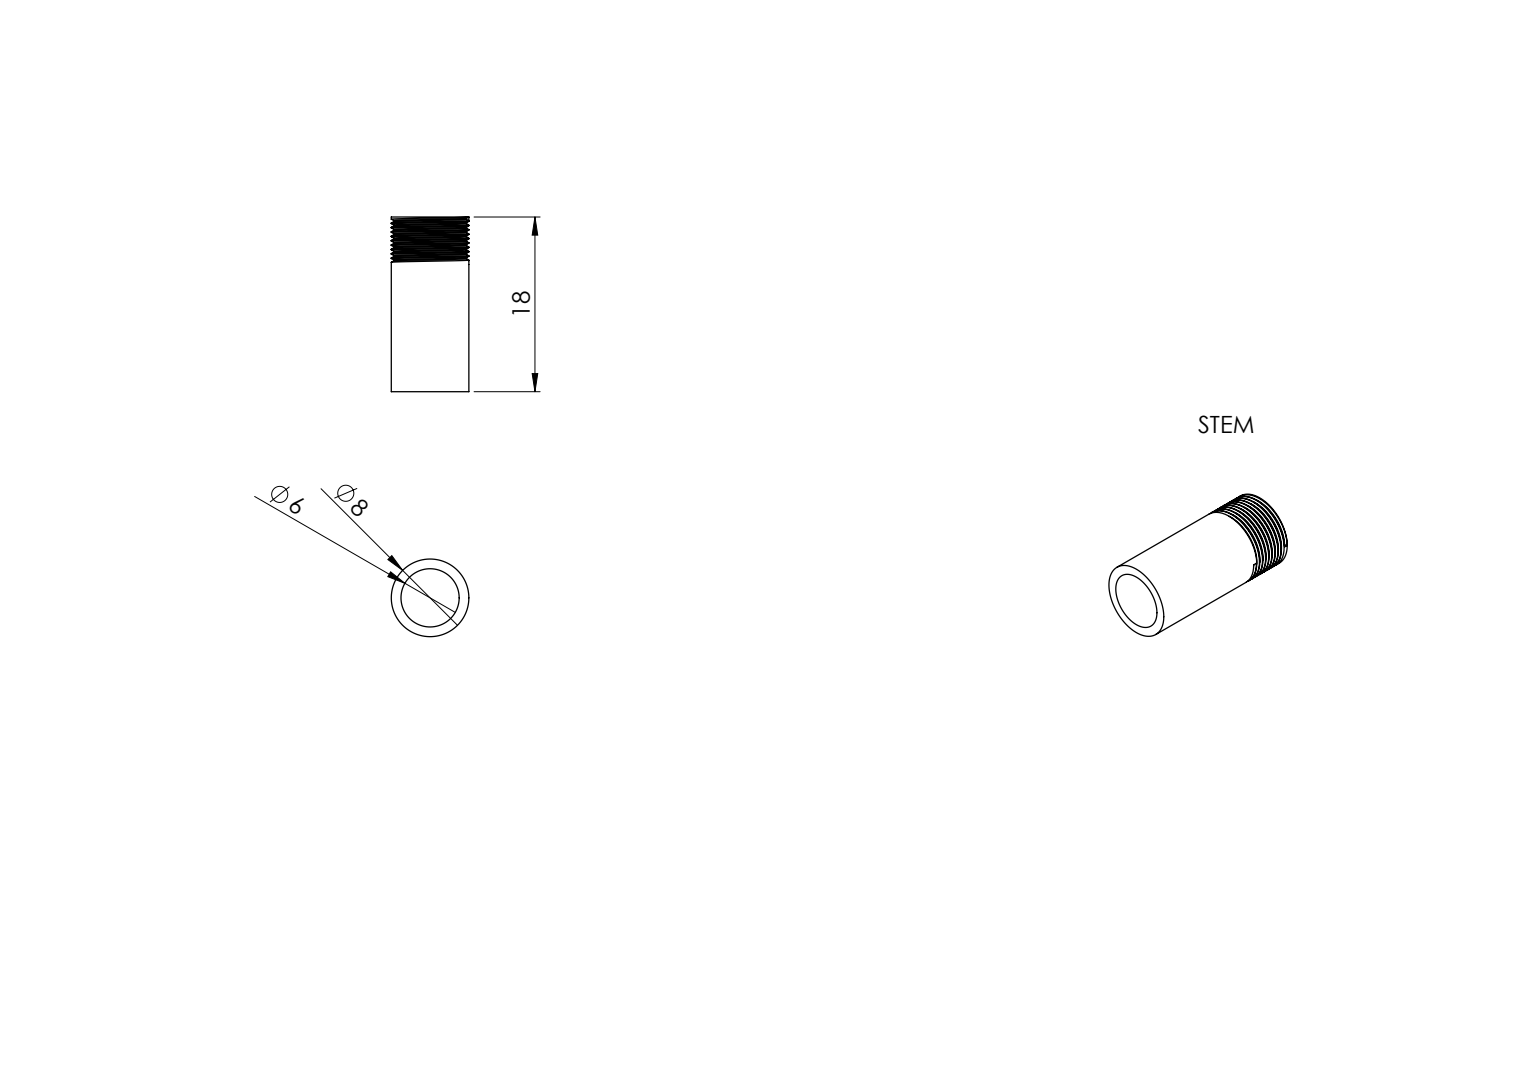
ISO-10303-21;
HEADER;
FILE_DESCRIPTION (('STEP AP214'),
    '1' );
FILE_NAME ('stem.step',
    '2026-10-26T12:50:16',
    ( '' ),
    ( '' ),
    'SwSTEP 2.0',
    'SolidWorks 2026',
    '' );
FILE_SCHEMA (( 'AUTOMOTIVE_DESIGN' ));
ENDSEC;

DATA;
#2=CARTESIAN_POINT ( 'NONE',  ( -3.756430356249997882, -11.16877607737301226, 2.653124999385483296 ) ) ;
#3=CARTESIAN_POINT ( 'NONE',  ( 2.000000000000003997, -5.535898384862238508, 4.518749998770967835 ) ) ;
#8=CARTESIAN_POINT ( 'NONE',  ( 4.000000000000003553, -8.999999999999992895, 1.743749998770967924 ) ) ;
#9=CARTESIAN_POINT ( 'NONE',  ( 2.620986760973688460E-15, -13.61880215351699874, 3.037499999999999201 ) ) ;
#11=CARTESIAN_POINT ( 'NONE',  ( 4.000000000000003553, -8.999999999999992895, 2.643749998770966059 ) ) ;
#36=CARTESIAN_POINT ( 'NONE',  ( 3.756430356250004099, -6.831223922626973533, 1.190624999385485383 ) ) ;
#74=( BOUNDED_CURVE ( )  B_SPLINE_CURVE ( 2, ( #2295, #21785, #5959, #10252, #8301, #13672, #11709 ),
 .UNSPECIFIED., .F., .F. ) 
 B_SPLINE_CURVE_WITH_KNOTS ( ( 3, 2, 2, 3 ),
 ( 0.8999999999999996891, 0.9166666666666665186, 0.9333333333333335702, 0.9500000000000003997 ),
 .UNSPECIFIED. ) 
 CURVE ( )  GEOMETRIC_REPRESENTATION_ITEM ( )  RATIONAL_B_SPLINE_CURVE ( ( 1.000000000000002665, 0.8660254037844360431, 1.000000000000000000, 0.8660254037844387076, 1.000000000000000000, 0.8660254037844351549, 1.000000000000003553 ) ) 
 REPRESENTATION_ITEM ( '' )  );
#103=CARTESIAN_POINT ( 'NONE',  ( 2.672651547586948120E-15, -13.33755215474603162, 2.278124999385481964 ) ) ;
#109=SHAPE_REPRESENTATION_RELATIONSHIP ( 'NONE' , 'NONE' ,  #19829, #5978 ) ;
#141=CARTESIAN_POINT ( 'NONE',  ( -3.756430356249997882, -11.16877607737301226, 4.453124999385482674 ) ) ;
#142=CARTESIAN_POINT ( 'NONE',  ( 1.878215178125004048, -5.746835883940462963, 0.3281249993854831737 ) ) ;
#162=EDGE_LOOP ( 'NONE', ( #20423, #8282, #5140, #7710 ) ) ;
#171=CARTESIAN_POINT ( 'NONE',  ( 1.878215178125000939, -12.25316411605952283, 3.778124999385484628 ) ) ;
#176=CARTESIAN_POINT ( 'NONE',  ( 3.756430356250003655, -8.999999999999992895, 0.5906249993854819635 ) ) ;
#227=CARTESIAN_POINT ( 'NONE',  ( -3.756430356249996994, -8.999999999999992895, 3.515624999385482674 ) ) ;
#266=CARTESIAN_POINT ( 'NONE',  ( -1.999999999999995781, -5.535898384862237620, 4.593749998770966236 ) ) ;
#277=ADVANCED_FACE ( 'NONE', ( #3080 ), #9085, .T. ) ;
#279=CARTESIAN_POINT ( 'NONE',  ( 3.999999999999994227, -11.30940107675849937, 1.762499999999997735 ) ) ;
#293=CARTESIAN_POINT ( 'NONE',  ( -3.756430356249996994, -8.999999999999992895, 2.728124999385482585 ) ) ;
#294=CARTESIAN_POINT ( 'NONE',  ( -1.999999999999995781, -5.535898384862237620, 1.443749998770966325 ) ) ;
#298=CARTESIAN_POINT ( 'NONE',  ( 1.878215178125000939, -12.25316411605952283, 0.9656249993854824076 ) ) ;
#337=VERTEX_POINT ( 'NONE', #16684 ) ;
#344=EDGE_CURVE ( 'NONE', #1313, #21005, #7390, .T. ) ;
#350=CARTESIAN_POINT ( 'NONE',  ( 1.878215178125000939, -12.25316411605952283, 4.565624999385481608 ) ) ;
#353=CARTESIAN_POINT ( 'NONE',  ( 3.752267015613588906E-15, -4.381197846482986158, 1.012499999999998401 ) ) ;
#392=CARTESIAN_POINT ( 'NONE',  ( 3.735045420075836212E-15, -4.662447845253954171, 2.165624999385483029 ) ) ;
#404=CARTESIAN_POINT ( 'NONE',  ( 4.000000000000003553, -8.999999999999992895, 2.700000000000001066 ) ) ;
#428=CARTESIAN_POINT ( 'NONE',  ( 3.756430356250002323, -11.16877607737301226, 1.565624999385482941 ) ) ;
#429=CARTESIAN_POINT ( 'NONE',  ( -4.000000000000033751, -6.690598923241509510, 1.481249998770963749 ) ) ;
#434=CARTESIAN_POINT ( 'NONE',  ( 1.878215178125004048, -5.746835883940462963, 1.565624999385482274 ) ) ;
#435=CARTESIAN_POINT ( 'NONE',  ( 2.000000000000003997, -5.535898384862238508, 3.675000000000001155 ) ) ;
#439=CARTESIAN_POINT ( 'NONE',  ( -1.878215178124998497, -12.25316411605951927, 1.003124999385485161 ) ) ;
#466=EDGE_CURVE ( 'NONE', #13776, #14884, #16423, .T. ) ;
#470=CARTESIAN_POINT ( 'NONE',  ( 4.000000000000003553, -8.999999999999992895, 0.1968749993854837510 ) ) ;
#523=VERTEX_POINT ( 'NONE', #23469 ) ;
#526=CARTESIAN_POINT ( 'NONE',  ( -1.999999999999995781, -5.535898384862237620, 1.950000000000000400 ) ) ;
#528=CARTESIAN_POINT ( 'NONE',  ( -3.756430356249997882, -11.16877607737301226, 3.215624999385481964 ) ) ;
#543=DIRECTION ( 'NONE',  ( 0.000000000000000000, 0.000000000000000000, 1.000000000000000000 ) ) ;
#561=CARTESIAN_POINT ( 'NONE',  ( -1.878215178124998497, -12.25316411605951927, 2.353124999385485694 ) ) ;
#568=CARTESIAN_POINT ( 'NONE',  ( 3.756430356250004099, -6.831223922626973533, 2.428124999385481431 ) ) ;
#573=CARTESIAN_POINT ( 'NONE',  ( -1.878215178124998497, -12.25316411605951927, 1.453124999385484228 ) ) ;
#574=FACE_OUTER_BOUND ( 'NONE', #3616, .T. ) ;
#586=CARTESIAN_POINT ( 'NONE',  ( 3.756430356250003655, -8.999999999999992895, 4.640624999385483562 ) ) ;
#651=CARTESIAN_POINT ( 'NONE',  ( 4.000000000000032863, -11.30940107675847983, 3.506249998770968102 ) ) ;
#652=CARTESIAN_POINT ( 'NONE',  ( 1.878215178125004048, -5.746835883940462963, 1.228124999385484584 ) ) ;
#668=CARTESIAN_POINT ( 'NONE',  ( -3.999999999999995559, -6.690598923241487306, 3.731249998770965970 ) ) ;
#669=ORIENTED_EDGE ( 'NONE', *, *, #3778, .F. ) ;
#677=ORIENTED_EDGE ( 'NONE', *, *, #7902, .T. ) ;
#682=CARTESIAN_POINT ( 'NONE',  ( 3.756430356250004099, -6.831223922626973533, 3.440624999385483829 ) ) ;
#686=DIRECTION ( 'NONE',  ( -0.000000000000000000, -0.000000000000000000, -1.000000000000000000 ) ) ;
#687=CARTESIAN_POINT ( 'NONE',  ( -3.999999999999953371, -6.690598923241463325, 0.6374999999999958478 ) ) ;
#689=CARTESIAN_POINT ( 'NONE',  ( -1.878215178124998497, -12.25316411605951927, 0.8906249993854836733 ) ) ;
#694=CARTESIAN_POINT ( 'NONE',  ( -1.878215178124995832, -5.746835883940462963, 2.653124999385483740 ) ) ;
#702=VERTEX_POINT ( 'NONE', #9421 ) ;
#705=ORIENTED_EDGE ( 'NONE', *, *, #13948, .T. ) ;
#737=CARTESIAN_POINT ( 'NONE',  ( -3.999999999999996447, -8.999999999999992895, 1.125000000000000888 ) ) ;
#768=ADVANCED_FACE ( 'NONE', ( #3150 ), #24982, .T. ) ;
#770=CARTESIAN_POINT ( 'NONE',  ( -3.756430356249995661, -6.831223922626973533, 0.8906249993854814528 ) ) ;
#776=CARTESIAN_POINT ( 'NONE',  ( 3.469446951953614189E-15, -8.999999999999992895, 18.00000000000000000 ) ) ;
#792=AXIS2_PLACEMENT_3D ( 'NONE', #15459, #16816, #19491 ) ;
#798=DIRECTION ( 'NONE',  ( -0.000000000000000000, -0.000000000000000000, -1.000000000000000000 ) ) ;
#801=CARTESIAN_POINT ( 'NONE',  ( 2.672651547586948120E-15, -13.33755215474602984, 4.640624999385483562 ) ) ;
#808=CARTESIAN_POINT ( 'NONE',  ( -1.878215178124995832, -5.746835883940462963, 3.890624999385482674 ) ) ;
#811=CARTESIAN_POINT ( 'NONE',  ( -1.999999999999995781, -5.535898384862237620, 3.750000000000000000 ) ) ;
#814=CARTESIAN_POINT ( 'NONE',  ( -3.756430356249996105, -6.831223922626973533, 3.140624999385484006 ) ) ;
#834=AXIS2_PLACEMENT_3D ( 'NONE', #5383, #9320, #12752 ) ;
#856=ORIENTED_EDGE ( 'NONE', *, *, #17515, .T. ) ;
#860=CARTESIAN_POINT ( 'NONE',  ( 3.999999999999956035, -11.30940107675852602, 4.406249998770962684 ) ) ;
#861=ORIENTED_EDGE ( 'NONE', *, *, #11086, .T. ) ;
#908=CARTESIAN_POINT ( 'NONE',  ( -3.756430356249995661, -6.831223922626973533, 1.790624999385484806 ) ) ;
#917=DIRECTION ( 'NONE',  ( 0.8660254037844397068, 0.000000000000000000, -0.4999999999999983347 ) ) ;
#921=LINE ( 'NONE', #7050, #24021 ) ;
#927=ORIENTED_EDGE ( 'NONE', *, *, #22382, .F. ) ;
#934=ORIENTED_EDGE ( 'NONE', *, *, #15408, .T. ) ;
#945=CARTESIAN_POINT ( 'NONE',  ( -3.756430356249996994, -8.999999999999992895, 0.3656249993854825409 ) ) ;
#951=CARTESIAN_POINT ( 'NONE',  ( 1.878215178125004048, -5.746835883940462963, 3.365624999385481875 ) ) ;
#953=CARTESIAN_POINT ( 'NONE',  ( -3.999999999999997335, -11.30940107675849404, 3.862499999999996714 ) ) ;
#988=CARTESIAN_POINT ( 'NONE',  ( 3.756430356250004099, -6.831223922626973533, 0.1781249993854828739 ) ) ;
#1034=CARTESIAN_POINT ( 'NONE',  ( -1.878215178124995832, -5.746835883940462963, 4.003124999385484273 ) ) ;
#1065=CARTESIAN_POINT ( 'NONE',  ( 3.756430356250002323, -11.16877607737301226, 0.5531249993854806535 ) ) ;
#1070=CARTESIAN_POINT ( 'NONE',  ( 2.620986760973688460E-15, -13.61880215351699874, 0.3375000000000008549 ) ) ;
#1074=DIRECTION ( 'NONE',  ( 0.000000000000000000, 0.000000000000000000, -1.000000000000000000 ) ) ;
#1075=CARTESIAN_POINT ( 'NONE',  ( -1.878215178124995832, -5.746835883940462963, 4.453124999385483562 ) ) ;
#1079=ORIENTED_EDGE ( 'NONE', *, *, #19912, .F. ) ;
#1091=DIRECTION ( 'NONE',  ( -0.000000000000000000, -0.000000000000000000, -1.000000000000000000 ) ) ;
#1108=EDGE_LOOP ( 'NONE', ( #16463, #25740, #25010, #7826 ) ) ;
#1148=CARTESIAN_POINT ( 'NONE',  ( -3.756430356249997438, -11.16877607737301048, 0.8531249993854844726 ) ) ;
#1155=LINE ( 'NONE', #20782, #4194 ) ;
#1181=CARTESIAN_POINT ( 'NONE',  ( 1.878215178125004048, -5.746835883940462963, 4.378124999385484273 ) ) ;
#1182=CARTESIAN_POINT ( 'NONE',  ( 2.000000000000003997, -5.535898384862238508, 1.818749998770966769 ) ) ;
#1188=CARTESIAN_POINT ( 'NONE',  ( 3.756430356250002323, -11.16877607737301226, 4.603124999385482141 ) ) ;
#1194=CARTESIAN_POINT ( 'NONE',  ( 3.756430356250003211, -6.831223922626973533, 3.890624999385483562 ) ) ;
#1197=VECTOR ( 'NONE', #3668, 1000.000000000000000 ) ;
#1201=ORIENTED_EDGE ( 'NONE', *, *, #18891, .T. ) ;
#1209=( BOUNDED_CURVE ( )  B_SPLINE_CURVE ( 2, ( #19108, #17166, #3281, #7221, #15205, #23173, #11254 ),
 .UNSPECIFIED., .F., .F. ) 
 B_SPLINE_CURVE_WITH_KNOTS ( ( 3, 2, 2, 3 ),
 ( 0.000000000000000000, 0.01666666666666663521, 0.03333333333333327042, 0.04999999999999990563 ),
 .UNSPECIFIED. ) 
 CURVE ( )  GEOMETRIC_REPRESENTATION_ITEM ( )  RATIONAL_B_SPLINE_CURVE ( ( 1.000000000000000000, 0.8660254037844387076, 1.000000000000000000, 0.8660254037844387076, 1.000000000000000000, 0.8660254037844394848, 0.9999999999999992228 ) ) 
 REPRESENTATION_ITEM ( '' )  );
#1218=VECTOR ( 'NONE', #19343, 1000.000000000000000 ) ;
#1283=CARTESIAN_POINT ( 'NONE',  ( -3.756430356249996105, -6.831223922626973533, 0.7781249993854825187 ) ) ;
#1285=AXIS2_PLACEMENT_3D ( 'NONE', #1608, #11806, #20026 ) ;
#1313=VERTEX_POINT ( 'NONE', #11561 ) ;
#1323=CARTESIAN_POINT ( 'NONE',  ( 1.878215178125004048, -5.746835883940462963, 1.565624999385482274 ) ) ;
#1324=CARTESIAN_POINT ( 'NONE',  ( -1.999999999999995781, -5.535898384862237620, 1.443749998770966325 ) ) ;
#1332=CARTESIAN_POINT ( 'NONE',  ( -1.878215178124995832, -5.746835883940462963, 2.990624999385481431 ) ) ;
#1334=LINE ( 'NONE', #11391, #10437 ) ;
#1340=CARTESIAN_POINT ( 'NONE',  ( 3.756430356250003211, -6.831223922626973533, 3.440624999385483829 ) ) ;
#1403=CARTESIAN_POINT ( 'NONE',  ( 4.000000000000003553, -8.999999999999992895, 3.093749998770968457 ) ) ;
#1417=EDGE_LOOP ( 'NONE', ( #18226, #25662, #5734, #10746 ) ) ;
#1420=CARTESIAN_POINT ( 'NONE',  ( 3.735045420075836212E-15, -4.662447845253954171, 2.053124999385483651 ) ) ;
#1422=ADVANCED_FACE ( 'NONE', ( #24079 ), #8392, .F. ) ;
#1445=VERTEX_POINT ( 'NONE', #14802 ) ;
#1453=CARTESIAN_POINT ( 'NONE',  ( -3.756430356249995661, -6.831223922626973533, 2.578124999385481342 ) ) ;
#1454=CARTESIAN_POINT ( 'NONE',  ( 4.000000000000003553, -8.999999999999992895, 2.643749998770966059 ) ) ;
#1459=CARTESIAN_POINT ( 'NONE',  ( 2.000000000000000888, -12.46410161513774817, 2.174999999999999822 ) ) ;
#1464=CARTESIAN_POINT ( 'NONE',  ( 2.672651547586948120E-15, -13.33755215474603162, 4.190624999385483385 ) ) ;
#1485=CARTESIAN_POINT ( 'NONE',  ( 3.469446951953614189E-15, -8.999999999999992895, 18.00000000000000000 ) ) ;
#1502=CARTESIAN_POINT ( 'NONE',  ( 4.000000000000049738, -6.690598923241514839, 4.087499999999997691 ) ) ;
#1536=EDGE_CURVE ( 'NONE', #4330, #17764, #6946, .T. ) ;
#1542=CARTESIAN_POINT ( 'NONE',  ( 3.735045420075836212E-15, -4.662447845253954171, 3.965624999385486404 ) ) ;
#1558=ORIENTED_EDGE ( 'NONE', *, *, #2307, .F. ) ;
#1572=CARTESIAN_POINT ( 'NONE',  ( 1.878215178125004048, -5.746835883940462963, 2.015624999385484450 ) ) ;
#1573=CARTESIAN_POINT ( 'NONE',  ( 2.620986760973688460E-15, -13.61880215351699874, 1.181249998770967258 ) ) ;
#1578=CARTESIAN_POINT ( 'NONE',  ( 4.000000000000003553, -8.999999999999992895, 1.799999999999999600 ) ) ;
#1589=CARTESIAN_POINT ( 'NONE',  ( 4.000000000000003553, -8.999999999999992895, 3.993749998770966592 ) ) ;
#1608=CARTESIAN_POINT ( 'NONE',  ( 3.469446951953614189E-15, -8.999999999999992895, 18.00000000000000000 ) ) ;
#1670=CARTESIAN_POINT ( 'NONE',  ( -3.756430356249997438, -11.16877607737301048, 0.4031249993854806868 ) ) ;
#1688=EDGE_CURVE ( 'NONE', #1445, #19775, #10234, .T. ) ;
#1689=CARTESIAN_POINT ( 'NONE',  ( 4.000000000000034639, -6.690598923241508622, 2.287499999999995648 ) ) ;
#1691=DIRECTION ( 'NONE',  ( 0.000000000000000000, 0.000000000000000000, 1.000000000000000000 ) ) ;
#1710=CARTESIAN_POINT ( 'NONE',  ( -3.756430356249996994, -8.999999999999992895, 3.965624999385481519 ) ) ;
#1711=CARTESIAN_POINT ( 'NONE',  ( -1.999999999999995781, -5.535898384862237620, 0.9937499987709673688 ) ) ;
#1717=CARTESIAN_POINT ( 'NONE',  ( 4.000000000000003553, -6.690598923241489970, 1.387499999999999956 ) ) ;
#1747=CARTESIAN_POINT ( 'NONE',  ( 3.469446951953614189E-15, -8.999999999999992895, 18.00000000000000000 ) ) ;
#1756=CARTESIAN_POINT ( 'NONE',  ( -1.878215178124995832, -5.746835883940462963, 0.4031249993854852942 ) ) ;
#1770=VERTEX_POINT ( 'NONE', #6410 ) ;
#1772=CARTESIAN_POINT ( 'NONE',  ( -4.000000000000057732, -6.690598923241522833, 4.237499999999998934 ) ) ;
#1792=ORIENTED_EDGE ( 'NONE', *, *, #11977, .T. ) ;
#1808=CARTESIAN_POINT ( 'NONE',  ( 1.878215178125004048, -5.746835883940462963, 2.915624999385482585 ) ) ;
#1839=EDGE_CURVE ( 'NONE', #12074, #6033, #921, .T. ) ;
#1845=CARTESIAN_POINT ( 'NONE',  ( -3.756430356249995661, -6.831223922626973533, 3.478124999385480809 ) ) ;
#1846=CARTESIAN_POINT ( 'NONE',  ( 3.735045420075836212E-15, -4.662447845253954171, 0.8156249993854834957 ) ) ;
#1851=CARTESIAN_POINT ( 'NONE',  ( 3.752267015613588906E-15, -4.381197846482986158, 2.362499999999997602 ) ) ;
#1861=DIRECTION ( 'NONE',  ( 0.000000000000000000, 0.000000000000000000, -1.000000000000000000 ) ) ;
#1864=DIRECTION ( 'NONE',  ( 1.000000000000000000, 0.000000000000000000, 0.000000000000000000 ) ) ;
#1875=CARTESIAN_POINT ( 'NONE',  ( 3.735045420075836212E-15, -4.662447845253954171, 0.3656249993854837066 ) ) ;
#1893=ORIENTED_EDGE ( 'NONE', *, *, #23260, .F. ) ;
#1904=( BOUNDED_CURVE ( )  B_SPLINE_CURVE ( 2, ( #10676, #20494, #20632, #22333, #12389, #4415, #20108 ),
 .UNSPECIFIED., .F., .F. ) 
 B_SPLINE_CURVE_WITH_KNOTS ( ( 3, 2, 2, 3 ),
 ( 0.2500000000000002776, 0.2666666666666669405, 0.2833333333333335480, 0.3000000000000002109 ),
 .UNSPECIFIED. ) 
 CURVE ( )  GEOMETRIC_REPRESENTATION_ITEM ( )  RATIONAL_B_SPLINE_CURVE ( ( 0.9999999999999977796, 0.8660254037844409281, 1.000000000000000000, 0.8660254037844387076, 1.000000000000000000, 0.8660254037844369313, 1.000000000000001776 ) ) 
 REPRESENTATION_ITEM ( '' )  );
#1929=CARTESIAN_POINT ( 'NONE',  ( 3.756430356250003211, -6.831223922626973533, 4.228124999385484806 ) ) ;
#1932=CARTESIAN_POINT ( 'NONE',  ( -4.000000000000012434, -11.30940107675848516, 3.862499999999996714 ) ) ;
#1960=CARTESIAN_POINT ( 'NONE',  ( 3.756430356250004099, -6.831223922626973533, 3.778124999385480631 ) ) ;
#1961=CARTESIAN_POINT ( 'NONE',  ( 2.000000000000000888, -12.46410161513774817, 3.468749998770968901 ) ) ;
#1967=CARTESIAN_POINT ( 'NONE',  ( 4.000000000000003553, -8.999999999999992895, 1.350000000000000533 ) ) ;
#1978=CARTESIAN_POINT ( 'NONE',  ( 4.000000000000003553, -8.999999999999992895, 4.696874999385483918 ) ) ;
#1990=CARTESIAN_POINT ( 'NONE',  ( 1.878215178125000939, -12.25316411605952283, 1.078124999385483784 ) ) ;
#2046=DIRECTION ( 'NONE',  ( -0.000000000000000000, -0.000000000000000000, -1.000000000000000000 ) ) ;
#2051=( BOUNDED_CURVE ( )  B_SPLINE_CURVE ( 2, ( #6648, #14634, #22615, #4703, #10569, #651, #16728 ),
 .UNSPECIFIED., .F., .F. ) 
 B_SPLINE_CURVE_WITH_KNOTS ( ( 3, 2, 2, 3 ),
 ( 0.6500000000000002442, 0.6666666666666668517, 0.6833333333333335702, 0.7000000000000001776 ),
 .UNSPECIFIED. ) 
 CURVE ( )  GEOMETRIC_REPRESENTATION_ITEM ( )  RATIONAL_B_SPLINE_CURVE ( ( 0.9999999999999982236, 0.8660254037844404840, 1.000000000000000000, 0.8660254037844387076, 1.000000000000000000, 0.8660254037844369313, 1.000000000000001776 ) ) 
 REPRESENTATION_ITEM ( '' )  );
#2053=VECTOR ( 'NONE', #21376, 1000.000000000000000 ) ;
#2055=CARTESIAN_POINT ( 'NONE',  ( 3.756430356250002323, -11.16877607737301403, 4.153124999385482852 ) ) ;
#2059=CARTESIAN_POINT ( 'NONE',  ( 2.620986760973688460E-15, -13.61880215351699874, 3.937499999999998224 ) ) ;
#2070=CARTESIAN_POINT ( 'NONE',  ( -1.999999999999995781, -5.535898384862237620, 2.399999999999999467 ) ) ;
#2091=CARTESIAN_POINT ( 'NONE',  ( 1.878215178125000939, -12.25316411605952283, 4.115624999385482319 ) ) ;
#2092=CARTESIAN_POINT ( 'NONE',  ( -1.999999999999998224, -12.46410161513774639, 4.293749998770968190 ) ) ;
#2104=VECTOR ( 'NONE', #14071, 1000.000000000000000 ) ;
#2114=CYLINDRICAL_SURFACE ( 'NONE', #6645, 4.000000000000000000 ) ;
#2118=CARTESIAN_POINT ( 'NONE',  ( 2.000000000000003997, -5.535898384862238508, 2.718749998770968013 ) ) ;
#2134=CARTESIAN_POINT ( 'NONE',  ( -1.878215178124998497, -12.25316411605951927, 1.790624999385481697 ) ) ;
#2142=ORIENTED_EDGE ( 'NONE', *, *, #19912, .T. ) ;
#2148=CARTESIAN_POINT ( 'NONE',  ( 4.000000000000003553, -8.999999999999992895, 0.3937499987709675020 ) ) ;
#2174=LINE ( 'NONE', #10135, #11663 ) ;
#2191=CARTESIAN_POINT ( 'NONE',  ( -1.878215178124995832, -5.746835883940462963, 2.090624999385483296 ) ) ;
#2196=CARTESIAN_POINT ( 'NONE',  ( 3.999999999999956035, -11.30940107675852602, 4.012499999999995737 ) ) ;
#2225=EDGE_CURVE ( 'NONE', #11292, #18617, #20028, .T. ) ;
#2227=CARTESIAN_POINT ( 'NONE',  ( -1.878215178124995832, -5.746835883940462963, 4.340624999385481964 ) ) ;
#2228=CARTESIAN_POINT ( 'NONE',  ( -1.999999999999995781, -5.535898384862237620, 3.693749998770968546 ) ) ;
#2258=CARTESIAN_POINT ( 'NONE',  ( 3.756430356250002323, -11.16877607737301226, 2.015624999385483118 ) ) ;
#2264=CARTESIAN_POINT ( 'NONE',  ( 3.756430356250003655, -8.999999999999992895, 2.390624999385481342 ) ) ;
#2267=CARTESIAN_POINT ( 'NONE',  ( 3.469446951953614189E-15, -8.999999999999992895, 0.000000000000000000 ) ) ;
#2270=FACE_OUTER_BOUND ( 'NONE', #11908, .T. ) ;
#2276=ORIENTED_EDGE ( 'NONE', *, *, #7804, .F. ) ;
#2295=CARTESIAN_POINT ( 'NONE',  ( 4.000000000000003553, -8.999999999999992895, 4.443749998770965881 ) ) ;
#2307=EDGE_CURVE ( 'NONE', #20603, #13396, #13885, .T. ) ;
#2315=CARTESIAN_POINT ( 'NONE',  ( 3.756430356250003211, -6.831223922626973533, 3.778124999385480631 ) ) ;
#2332=ORIENTED_EDGE ( 'NONE', *, *, #22414, .T. ) ;
#2342=PRODUCT_DEFINITION_SHAPE ( 'NONE', 'NONE',  #17659 ) ;
#2348=CARTESIAN_POINT ( 'NONE',  ( 2.672651547586948120E-15, -13.33755215474602984, 4.078124999385480010 ) ) ;
#2349=CARTESIAN_POINT ( 'NONE',  ( 3.756430356250003655, -8.999999999999992895, 0.7031249993854835623 ) ) ;
#2360=CARTESIAN_POINT ( 'NONE',  ( 3.999999999999942268, -6.690598923241455331, 2.737500000000000266 ) ) ;
#2372=VERTEX_POINT ( 'NONE', #20006 ) ;
#2379=CARTESIAN_POINT ( 'NONE',  ( 3.735045420075836212E-15, -4.662447845253954171, 2.615624999385482319 ) ) ;
#2380=CARTESIAN_POINT ( 'NONE',  ( 3.752267015613588906E-15, -4.381197846482986158, 1.406249998770964904 ) ) ;
#2384=CARTESIAN_POINT ( 'NONE',  ( 3.756430356250002323, -11.16877607737301226, 1.003124999385480276 ) ) ;
#2387=CARTESIAN_POINT ( 'NONE',  ( 3.756430356250002323, -11.16877607737301403, 2.015624999385483118 ) ) ;
#2426=ORIENTED_EDGE ( 'NONE', *, *, #22750, .F. ) ;
#2458=ORIENTED_EDGE ( 'NONE', *, *, #23613, .T. ) ;
#2467=CARTESIAN_POINT ( 'NONE',  ( 3.756430356250004099, -6.831223922626973533, 2.540624999385480809 ) ) ;
#2490=ORIENTED_EDGE ( 'NONE', *, *, #11535, .T. ) ;
#2500=ORIENTED_EDGE ( 'NONE', *, *, #20767, .T. ) ;
#2506=CARTESIAN_POINT ( 'NONE',  ( 3.756430356250004099, -6.831223922626973533, 2.540624999385480809 ) ) ;
#2512=CARTESIAN_POINT ( 'NONE',  ( 1.878215178125004048, -5.746835883940462963, 2.015624999385484450 ) ) ;
#2516=CARTESIAN_POINT ( 'NONE',  ( -3.756430356249996105, -6.831223922626973533, 0.8906249993854813418 ) ) ;
#2518=DIRECTION ( 'NONE',  ( -0.000000000000000000, -0.000000000000000000, -1.000000000000000000 ) ) ;
#2545=CARTESIAN_POINT ( 'NONE',  ( -3.999999999999996447, -8.999999999999992895, 2.024999999999999023 ) ) ;
#2589=EDGE_CURVE ( 'NONE', #13396, #21005, #14278, .T. ) ;
#2612=CARTESIAN_POINT ( 'NONE',  ( 1.878215178125000939, -12.25316411605952283, 1.978124999385485250 ) ) ;
#2620=CARTESIAN_POINT ( 'NONE',  ( -3.999999999999953371, -6.690598923241463325, 1.031249998770966458 ) ) ;
#2623=CARTESIAN_POINT ( 'NONE',  ( 4.000000000000003553, -8.999999999999992895, 3.149999999999999911 ) ) ;
#2644=CARTESIAN_POINT ( 'NONE',  ( -1.878215178124995832, -5.746835883940462963, 3.103124999385483029 ) ) ;
#2649=CARTESIAN_POINT ( 'NONE',  ( 1.878215178125004048, -5.746835883940462963, 2.915624999385482585 ) ) ;
#2651=CARTESIAN_POINT ( 'NONE',  ( 2.000000000000003997, -5.535898384862238508, 3.224999999999998757 ) ) ;
#2654=CARTESIAN_POINT ( 'NONE',  ( 3.756430356250003211, -6.831223922626973533, 2.540624999385480809 ) ) ;
#2655=CARTESIAN_POINT ( 'NONE',  ( 3.469446951953614189E-15, -8.999999999999992895, 0.000000000000000000 ) ) ;
#2693=CARTESIAN_POINT ( 'NONE',  ( -3.999999999999996447, -8.999999999999992895, 4.218749998770966236 ) ) ;
#2731=( BOUNDED_CURVE ( )  B_SPLINE_CURVE ( 2, ( #15582, #17410, #19227, #9428, #25373, #9546, #15446 ),
 .UNSPECIFIED., .F., .F. ) 
 B_SPLINE_CURVE_WITH_KNOTS ( ( 3, 2, 2, 3 ),
 ( 0.7500000000000000000, 0.7666666666666667185, 0.7833333333333332149, 0.7999999999999999334 ),
 .UNSPECIFIED. ) 
 CURVE ( )  GEOMETRIC_REPRESENTATION_ITEM ( )  RATIONAL_B_SPLINE_CURVE ( ( 1.000000000000000000, 0.8660254037844387076, 1.000000000000000000, 0.8660254037844387076, 1.000000000000000000, 0.8660254037844395958, 0.9999999999999991118 ) ) 
 REPRESENTATION_ITEM ( '' )  );
#2732=CARTESIAN_POINT ( 'NONE',  ( -3.756430356249995661, -6.831223922626973533, 2.690624999385480276 ) ) ;
#2763=CARTESIAN_POINT ( 'NONE',  ( 1.878215178125000939, -12.25316411605952283, 3.328124999385485783 ) ) ;
#2769=CARTESIAN_POINT ( 'NONE',  ( 3.756430356250003655, -8.999999999999992895, 3.290624999385483029 ) ) ;
#2771=CARTESIAN_POINT ( 'NONE',  ( 2.620986760973688460E-15, -13.61880215351699874, 3.487499999999998934 ) ) ;
#2774=CARTESIAN_POINT ( 'NONE',  ( 1.878215178125004048, -5.746835883940462963, 3.028124999385484184 ) ) ;
#2785=ORIENTED_EDGE ( 'NONE', *, *, #3875, .T. ) ;
#2799=CARTESIAN_POINT ( 'NONE',  ( 2.000000000000003997, -5.535898384862238508, 3.168749998770967302 ) ) ;
#2800=LINE ( 'NONE', #470, #5913 ) ;
#2813=CARTESIAN_POINT ( 'NONE',  ( 4.000000000000003553, -8.999999999999992895, 4.443749998770965881 ) ) ;
#2853=CARTESIAN_POINT ( 'NONE',  ( -3.999999999999973355, -6.690598923241474871, 1.987499999999999600 ) ) ;
#2855=CARTESIAN_POINT ( 'NONE',  ( 3.735045420075836212E-15, -4.662447845253954171, 2.615624999385482319 ) ) ;
#2887=( BOUNDED_CURVE ( )  B_SPLINE_CURVE ( 2, ( #25233, #21300, #21053, #8899, #8753, #5098, #6922 ),
 .UNSPECIFIED., .F., .F. ) 
 B_SPLINE_CURVE_WITH_KNOTS ( ( 3, 2, 2, 3 ),
 ( 0.04999999999999990563, 0.06666666666666654084, 0.08333333333333316217, 0.09999999999999981126 ),
 .UNSPECIFIED. ) 
 CURVE ( )  GEOMETRIC_REPRESENTATION_ITEM ( )  RATIONAL_B_SPLINE_CURVE ( ( 1.000000000000000666, 0.8660254037844378194, 1.000000000000000000, 0.8660254037844387076, 1.000000000000000000, 0.8660254037844402619, 0.9999999999999984457 ) ) 
 REPRESENTATION_ITEM ( '' )  );
#2889=CARTESIAN_POINT ( 'NONE',  ( 1.878215178125004048, -5.746835883940462963, 3.928124999385485872 ) ) ;
#2895=CARTESIAN_POINT ( 'NONE',  ( 4.000000000000001776, -11.30940107675849760, 0.4124999999999987566 ) ) ;
#2901=CARTESIAN_POINT ( 'NONE',  ( 3.756430356250003211, -6.831223922626973533, 2.090624999385480631 ) ) ;
#2937=FACE_OUTER_BOUND ( 'NONE', #17685, .T. ) ;
#2945=ORIENTED_EDGE ( 'NONE', *, *, #12834, .T. ) ;
#2992=EDGE_CURVE ( 'NONE', #9030, #7533, #16678, .T. ) ;
#2995=CARTESIAN_POINT ( 'NONE',  ( 3.756430356250003655, -8.999999999999992895, 2.503124999385482941 ) ) ;
#3031=CARTESIAN_POINT ( 'NONE',  ( -3.756430356249996994, -8.999999999999992895, 0.8156249993854814972 ) ) ;
#3037=CARTESIAN_POINT ( 'NONE',  ( 3.756430356250003655, -8.999999999999992895, 3.740624999385481875 ) ) ;
#3038=DIRECTION ( 'NONE',  ( -1.000000000000000000, 0.000000000000000000, 0.000000000000000000 ) ) ;
#3039=CARTESIAN_POINT ( 'NONE',  ( 4.000000000000003553, -6.690598923241489970, 3.187499999999998668 ) ) ;
#3041=CARTESIAN_POINT ( 'NONE',  ( 2.672651547586948120E-15, -13.33755215474603162, 3.290624999385483918 ) ) ;
#3056=CARTESIAN_POINT ( 'NONE',  ( -3.999999999999996447, -8.999999999999992895, 2.474999999999997868 ) ) ;
#3060=CYLINDRICAL_SURFACE ( 'NONE', #17949, 4.000000000000000000 ) ;
#3080=FACE_OUTER_BOUND ( 'NONE', #12480, .T. ) ;
#3116=ORIENTED_EDGE ( 'NONE', *, *, #19511, .F. ) ;
#3150=FACE_OUTER_BOUND ( 'NONE', #23571, .T. ) ;
#3152=CARTESIAN_POINT ( 'NONE',  ( 1.878215178125000939, -12.25316411605952283, 4.678124999385483207 ) ) ;
#3153=CARTESIAN_POINT ( 'NONE',  ( 2.000000000000000888, -12.46410161513774817, 1.218749998770966902 ) ) ;
#3156=CARTESIAN_POINT ( 'NONE',  ( 4.000000000000003553, -8.999999999999992895, 0.4499999999999990119 ) ) ;
#3194=ORIENTED_EDGE ( 'NONE', *, *, #19749, .T. ) ;
#3195=EDGE_LOOP ( 'NONE', ( #3439, #10877, #17181, #18667 ) ) ;
#3197=DIRECTION ( 'NONE',  ( -1.000000000000000000, 0.000000000000000000, 0.000000000000000000 ) ) ;
#3248=CARTESIAN_POINT ( 'NONE',  ( 4.000000000000003553, -8.999999999999992895, 18.00000000000000000 ) ) ;
#3252=CARTESIAN_POINT ( 'NONE',  ( 4.000000000000063061, -11.30940107675846207, 2.662499999999998757 ) ) ;
#3268=CARTESIAN_POINT ( 'NONE',  ( 3.756430356250003655, -8.999999999999992895, 1.490624999385483429 ) ) ;
#3269=CARTESIAN_POINT ( 'NONE',  ( 4.000000000000001776, -11.30940107675849760, 0.8062499987709654814 ) ) ;
#3275=CARTESIAN_POINT ( 'NONE',  ( 4.000000000000003553, -6.690598923241489970, 0.03749999999999697325 ) ) ;
#3281=CARTESIAN_POINT ( 'NONE',  ( 2.000000000000003997, -5.535898384862238508, 0.4687499987709661808 ) ) ;
#3317=ORIENTED_EDGE ( 'NONE', *, *, #16237, .T. ) ;
#3339=EDGE_CURVE ( 'NONE', #1770, #13208, #5711, .T. ) ;
#3367=CARTESIAN_POINT ( 'NONE',  ( -3.756430356249997438, -11.16877607737301048, 1.303124999385484095 ) ) ;
#3371=CARTESIAN_POINT ( 'NONE',  ( -3.756430356249997882, -11.16877607737301226, 4.115624999385481431 ) ) ;
#3405=CARTESIAN_POINT ( 'NONE',  ( -3.756430356249995661, -6.831223922626973533, 1.228124999385478144 ) ) ;
#3406=CARTESIAN_POINT ( 'NONE',  ( -1.999999999999998224, -12.46410161513774639, 1.593749998770967125 ) ) ;
#3411=CARTESIAN_POINT ( 'NONE',  ( -3.999999999999997335, -11.30940107675849404, 0.7124999999999986899 ) ) ;
#3417=( BOUNDED_CURVE ( )  B_SPLINE_CURVE ( 2, ( #11522, #11646, #23427, #19372, #9557, #5642, #24779 ),
 .UNSPECIFIED., .F., .F. ) 
 B_SPLINE_CURVE_WITH_KNOTS ( ( 3, 2, 2, 3 ),
 ( 0.9500000000000003997, 0.9666666666666670071, 0.9833333333333333925, 1.000000000000000000 ),
 .UNSPECIFIED. ) 
 CURVE ( )  GEOMETRIC_REPRESENTATION_ITEM ( )  RATIONAL_B_SPLINE_CURVE ( ( 0.9999999999999964473, 0.8660254037844422603, 1.000000000000000000, 0.8660254037844387076, 1.000000000000000000, 0.8660254037844387076, 1.000000000000000000 ) ) 
 REPRESENTATION_ITEM ( '' )  );
#3420=CARTESIAN_POINT ( 'NONE',  ( -1.878215178124998497, -12.25316411605951927, 3.703124999385482674 ) ) ;
#3437=AXIS2_PLACEMENT_3D ( 'NONE', #17377, #11597, #5215 ) ;
#3438=VECTOR ( 'NONE', #917, 999.9999999999998863 ) ;
#3439=ORIENTED_EDGE ( 'NONE', *, *, #16353, .F. ) ;
#3490=DIRECTION ( 'NONE',  ( 1.000000000000000000, 0.000000000000000000, 0.000000000000000000 ) ) ;
#3505=CARTESIAN_POINT ( 'NONE',  ( -1.878215178124995832, -5.746835883940462963, 1.640624999385484450 ) ) ;
#3506=CARTESIAN_POINT ( 'NONE',  ( -3.756430356249997882, -11.16877607737301226, 3.665624999385481697 ) ) ;
#3523=CARTESIAN_POINT ( 'NONE',  ( -3.999999999999996447, -8.999999999999992895, 2.474999999999997868 ) ) ;
#3536=CARTESIAN_POINT ( 'NONE',  ( -3.756430356249997882, -11.16877607737301226, 1.753124999385479832 ) ) ;
#3537=CARTESIAN_POINT ( 'NONE',  ( 2.000000000000003997, -5.535898384862238508, 1.368749998770967702 ) ) ;
#3541=CARTESIAN_POINT ( 'NONE',  ( -1.999999999999998224, -12.46410161513774639, 2.100000000000000977 ) ) ;
#3565=CARTESIAN_POINT ( 'NONE',  ( -3.756430356249995661, -6.831223922626973533, 0.8906249993854814528 ) ) ;
#3573=( BOUNDED_CURVE ( )  B_SPLINE_CURVE ( 2, ( #3523, #23653, #5731, #13711, #3774, #3252, #21829 ),
 .UNSPECIFIED., .F., .F. ) 
 B_SPLINE_CURVE_WITH_KNOTS ( ( 3, 2, 2, 3 ),
 ( 0.5499999999999997113, 0.5666666666666665408, 0.5833333333333335924, 0.6000000000000004219 ),
 .UNSPECIFIED. ) 
 CURVE ( )  GEOMETRIC_REPRESENTATION_ITEM ( )  RATIONAL_B_SPLINE_CURVE ( ( 1.000000000000002665, 0.8660254037844360431, 1.000000000000000000, 0.8660254037844387076, 1.000000000000000000, 0.8660254037844351549, 1.000000000000003553 ) ) 
 REPRESENTATION_ITEM ( '' )  );
#3593=ADVANCED_FACE ( 'NONE', ( #5590 ), #24012, .T. ) ;
#3610=CYLINDRICAL_SURFACE ( 'NONE', #18880, 3.000000000000000444 ) ;
#3616=EDGE_LOOP ( 'NONE', ( #1079, #18012, #11226, #20146 ) ) ;
#3623=CARTESIAN_POINT ( 'NONE',  ( -3.756430356249996994, -8.999999999999992895, 0.8156249993854814972 ) ) ;
#3625=CARTESIAN_POINT ( 'NONE',  ( -3.756430356249995661, -6.831223922626973533, 4.490624999385484095 ) ) ;
#3646=VERTEX_POINT ( 'NONE', #23747 ) ;
#3648=ORIENTED_EDGE ( 'NONE', *, *, #466, .T. ) ;
#3653=CARTESIAN_POINT ( 'NONE',  ( -3.756430356249995661, -6.831223922626973533, 3.928124999385480542 ) ) ;
#3654=CARTESIAN_POINT ( 'NONE',  ( 4.000000000000003553, -8.999999999999992895, 3.093749998770968457 ) ) ;
#3660=CARTESIAN_POINT ( 'NONE',  ( -3.999999999999997335, -11.30940107675849404, 1.162499999999998312 ) ) ;
#3667=CIRCLE ( 'NONE', #7007, 4.000000000000000000 ) ;
#3668=DIRECTION ( 'NONE',  ( -0.000000000000000000, -0.000000000000000000, -1.000000000000000000 ) ) ;
#3685=CARTESIAN_POINT ( 'NONE',  ( 3.756430356250004099, -6.831223922626973533, 0.7406249993854815417 ) ) ;
#3689=ADVANCED_FACE ( 'NONE', ( #16302 ), #12240, .F. ) ;
#3752=CARTESIAN_POINT ( 'NONE',  ( 2.672651547586948120E-15, -13.33755215474603162, 3.178124999385480987 ) ) ;
#3757=AXIS2_PLACEMENT_3D ( 'NONE', #8601, #22066, #24542 ) ;
#3759=CYLINDRICAL_SURFACE ( 'NONE', #23855, 4.000000000000000000 ) ;
#3774=CARTESIAN_POINT ( 'NONE',  ( 2.000000000000000888, -12.46410161513774817, 2.624999999999998668 ) ) ;
#3778=EDGE_CURVE ( 'NONE', #7533, #9331, #15068, .T. ) ;
#3791=CARTESIAN_POINT ( 'NONE',  ( 2.672651547586948120E-15, -13.33755215474602984, 2.278124999385481519 ) ) ;
#3792=CARTESIAN_POINT ( 'NONE',  ( -3.999999999999997335, -11.30940107675849404, 4.706249998770967835 ) ) ;
#3797=CARTESIAN_POINT ( 'NONE',  ( 4.000000000000003553, -8.999999999999992895, 2.249999999999998668 ) ) ;
#3799=CARTESIAN_POINT ( 'NONE',  ( 3.999999999999970690, -11.30940107675851536, 2.606249998770964194 ) ) ;
#3832=CARTESIAN_POINT ( 'NONE',  ( 2.672651547586948120E-15, -13.33755215474603162, 0.5906249993854857383 ) ) ;
#3848=EDGE_CURVE ( 'NONE', #10226, #10048, #18220, .T. ) ;
#3849=CARTESIAN_POINT ( 'NONE',  ( 3.752267015613588906E-15, -4.381197846482986158, 4.162500000000000533 ) ) ;
#3860=EDGE_CURVE ( 'NONE', #23657, #4330, #17268, .T. ) ;
#3869=CARTESIAN_POINT ( 'NONE',  ( 4.000000000000063061, -11.30940107675846207, 3.056249998770965259 ) ) ;
#3875=EDGE_CURVE ( 'NONE', #6033, #18161, #25068, .T. ) ;
#3889=CARTESIAN_POINT ( 'NONE',  ( -1.878215178124995832, -5.746835883940462963, 2.990624999385481431 ) ) ;
#3893=EDGE_CURVE ( 'NONE', #12074, #337, #1209, .T. ) ;
#3922=CARTESIAN_POINT ( 'NONE',  ( 3.756430356250004099, -6.831223922626973533, 2.878124999385481608 ) ) ;
#3923=CARTESIAN_POINT ( 'NONE',  ( -3.999999999999996003, -6.690598923241487306, 3.731249998770965970 ) ) ;
#3930=CARTESIAN_POINT ( 'NONE',  ( 2.000000000000000888, -12.46410161513774817, 2.624999999999998668 ) ) ;
#3932=DIRECTION ( 'NONE',  ( 0.000000000000000000, -1.000000000000000000, 0.000000000000000000 ) ) ;
#3946=CARTESIAN_POINT ( 'NONE',  ( 3.469446951953614189E-15, -8.999999999999992895, 0.000000000000000000 ) ) ;
#3952=CARTESIAN_POINT ( 'NONE',  ( -3.999999999999996447, -8.999999999999992895, 3.768749998770966947 ) ) ;
#3956=CARTESIAN_POINT ( 'NONE',  ( 3.756430356250004099, -6.831223922626973533, 0.2906249993854818081 ) ) ;
#3964=CARTESIAN_POINT ( 'NONE',  ( 3.756430356250002323, -11.16877607737301403, 0.6656249993854835845 ) ) ;
#4010=CARTESIAN_POINT ( 'NONE',  ( -3.756430356249996994, -8.999999999999992895, 4.415624999385483918 ) ) ;
#4013=CARTESIAN_POINT ( 'NONE',  ( -1.999999999999998224, -12.46410161513774639, 3.900000000000000799 ) ) ;
#4033=ORIENTED_EDGE ( 'NONE', *, *, #4034, .T. ) ;
#4034=EDGE_CURVE ( 'NONE', #25772, #10674, #25278, .T. ) ;
#4035=VERTEX_POINT ( 'NONE', #3952 ) ;
#4036=ORIENTED_EDGE ( 'NONE', *, *, #3848, .F. ) ;
#4042=CARTESIAN_POINT ( 'NONE',  ( 3.756430356250003655, -8.999999999999992895, 4.640624999385483562 ) ) ;
#4043=CARTESIAN_POINT ( 'NONE',  ( 2.620986760973688460E-15, -13.61880215351699874, 4.781249998770965348 ) ) ;
#4077=CARTESIAN_POINT ( 'NONE',  ( -1.878215178124995832, -5.746835883940462963, 1.640624999385484450 ) ) ;
#4091=CARTESIAN_POINT ( 'NONE',  ( 3.752267015613588906E-15, -4.381197846482986158, 2.306249998770968368 ) ) ;
#4102=CARTESIAN_POINT ( 'NONE',  ( 4.000000000000003553, -8.999999999999992895, 18.00000000000000000 ) ) ;
#4134=CARTESIAN_POINT ( 'NONE',  ( 3.735045420075836212E-15, -4.662447845253954171, 3.403124999385482408 ) ) ;
#4139=SURFACE_SIDE_STYLE ('',( #6368 ) ) ;
#4174=CARTESIAN_POINT ( 'NONE',  ( -3.756430356249997882, -11.16877607737301226, 0.5156249993854836733 ) ) ;
#4188=CARTESIAN_POINT ( 'NONE',  ( -3.999999999999982681, -11.30940107675850292, 1.612499999999998490 ) ) ;
#4194=VECTOR ( 'NONE', #16741, 1000.000000000000000 ) ;
#4206=CARTESIAN_POINT ( 'NONE',  ( 2.672651547586948120E-15, -13.33755215474602984, 1.490624999385481209 ) ) ;
#4210=AXIS2_PLACEMENT_3D ( 'NONE', #16704, #18929, #10671 ) ;
#4211=CARTESIAN_POINT ( 'NONE',  ( 3.469446951953614189E-15, -8.999999999999992895, 18.00000000000000000 ) ) ;
#4214=CARTESIAN_POINT ( 'NONE',  ( -3.756430356249995661, -6.831223922626973533, 1.678124999385481875 ) ) ;
#4229=CARTESIAN_POINT ( 'NONE',  ( 4.000000000000012434, -6.690598923241494411, 2.231249998770966858 ) ) ;
#4238=VECTOR ( 'NONE', #5982, 1000.000000000000000 ) ;
#4252=( BOUNDED_CURVE ( )  B_SPLINE_CURVE ( 2, ( #20654, #24839, #6794, #20374, #24959, #14899, #22872 ),
 .UNSPECIFIED., .F., .F. ) 
 B_SPLINE_CURVE_WITH_KNOTS ( ( 3, 2, 2, 3 ),
 ( 0.3000000000000002109, 0.3166666666666668184, 0.3333333333333334814, 0.3500000000000000888 ),
 .UNSPECIFIED. ) 
 CURVE ( )  GEOMETRIC_REPRESENTATION_ITEM ( )  RATIONAL_B_SPLINE_CURVE ( ( 0.9999999999999982236, 0.8660254037844404840, 1.000000000000000000, 0.8660254037844387076, 1.000000000000000000, 0.8660254037844378194, 1.000000000000000888 ) ) 
 REPRESENTATION_ITEM ( '' )  );
#4275=CARTESIAN_POINT ( 'NONE',  ( -3.756430356249996994, -8.999999999999992895, 2.615624999385480987 ) ) ;
#4276=CARTESIAN_POINT ( 'NONE',  ( -3.999999999999995559, -6.690598923241487306, 3.337499999999999023 ) ) ;
#4311=CARTESIAN_POINT ( 'NONE',  ( 3.756430356250004099, -6.831223922626973533, 0.2906249993854818081 ) ) ;
#4330=VERTEX_POINT ( 'NONE', #17285 ) ;
#4334=CARTESIAN_POINT ( 'NONE',  ( 4.000000000000034639, -6.690598923241508622, 2.681249998770965259 ) ) ;
#4340=CARTESIAN_POINT ( 'NONE',  ( 3.756430356250002323, -11.16877607737301226, 3.365624999385485872 ) ) ;
#4345=CARTESIAN_POINT ( 'NONE',  ( 3.756430356250002323, -11.16877607737301226, 2.353124999385479477 ) ) ;
#4348=CARTESIAN_POINT ( 'NONE',  ( 2.672651547586948120E-15, -13.33755215474603162, 1.040624999385485472 ) ) ;
#4357=CARTESIAN_POINT ( 'NONE',  ( 3.469446951953614189E-15, -8.999999999999992895, 0.000000000000000000 ) ) ;
#4387=CARTESIAN_POINT ( 'NONE',  ( 3.878215178125003604, -8.999999999999992895, 4.570312499692741781 ) ) ;
#4413=ORIENTED_EDGE ( 'NONE', *, *, #12834, .F. ) ;
#4415=CARTESIAN_POINT ( 'NONE',  ( 4.000000000000032863, -11.30940107675847983, 1.312499999999998890 ) ) ;
#4431=CARTESIAN_POINT ( 'NONE',  ( 3.752267015613588906E-15, -4.381197846482986158, 1.912500000000001865 ) ) ;
#4432=CARTESIAN_POINT ( 'NONE',  ( 3.756430356250004099, -6.831223922626973533, 1.640624999385484895 ) ) ;
#4440=CARTESIAN_POINT ( 'NONE',  ( -1.999999999999995781, -5.535898384862237620, 0.9937499987709673688 ) ) ;
#4461=CARTESIAN_POINT ( 'NONE',  ( 1.878215178125004048, -5.746835883940462963, 1.678124999385483651 ) ) ;
#4466=CARTESIAN_POINT ( 'NONE',  ( -1.878215178124998497, -12.25316411605951927, 2.690624999385483385 ) ) ;
#4468=CARTESIAN_POINT ( 'NONE',  ( 2.620986760973688460E-15, -13.61880215351699874, 3.937499999999998224 ) ) ;
#4471=CARTESIAN_POINT ( 'NONE',  ( 3.756430356250002323, -11.16877607737301403, 1.565624999385483163 ) ) ;
#4473=DIRECTION ( 'NONE',  ( 0.000000000000000000, 0.000000000000000000, 1.000000000000000000 ) ) ;
#4512=ORIENTED_EDGE ( 'NONE', *, *, #22869, .T. ) ;
#4519=CARTESIAN_POINT ( 'NONE',  ( 2.000000000000003997, -5.535898384862238508, 0.9750000000000001998 ) ) ;
#4523=CARTESIAN_POINT ( 'NONE',  ( 3.756430356250003655, -8.999999999999992895, 0.1406249993854830072 ) ) ;
#4556=CARTESIAN_POINT ( 'NONE',  ( 1.878215178125000939, -12.25316411605952283, 1.528124999385482852 ) ) ;
#4562=CARTESIAN_POINT ( 'NONE',  ( -3.999999999999980904, -6.690598923241480200, 3.787499999999999201 ) ) ;
#4567=CARTESIAN_POINT ( 'NONE',  ( 4.000000000000030198, -6.690598923241506846, 0.8812499987709628835 ) ) ;
#4593=CARTESIAN_POINT ( 'NONE',  ( -1.878215178124995832, -5.746835883940462963, 2.653124999385483740 ) ) ;
#4598=CARTESIAN_POINT ( 'NONE',  ( -3.756430356249995661, -6.831223922626973533, 2.578124999385481342 ) ) ;
#4600=CARTESIAN_POINT ( 'NONE',  ( 4.000000000000001776, -11.30940107675849760, 3.562499999999996891 ) ) ;
#4605=CARTESIAN_POINT ( 'NONE',  ( -3.756430356249997438, -11.16877607737301048, 0.9656249993854834068 ) ) ;
#4628=DIRECTION ( 'NONE',  ( -0.000000000000000000, -0.000000000000000000, -1.000000000000000000 ) ) ;
#4703=CARTESIAN_POINT ( 'NONE',  ( 2.620986760973688460E-15, -13.61880215351699874, 3.431249998770965703 ) ) ;
#4706=CARTESIAN_POINT ( 'NONE',  ( 1.878215178125000939, -12.25316411605952283, 1.078124999385483784 ) ) ;
#4717=CARTESIAN_POINT ( 'NONE',  ( 2.000000000000003997, -5.535898384862238508, 0.9187499987709686344 ) ) ;
#4740=CARTESIAN_POINT ( 'NONE',  ( 3.756430356250004099, -6.831223922626973533, 1.640624999385484895 ) ) ;
#4748=CARTESIAN_POINT ( 'NONE',  ( -3.756430356249996994, -8.999999999999992895, 4.415624999385483918 ) ) ;
#4750=CARTESIAN_POINT ( 'NONE',  ( -1.999999999999998224, -12.46410161513774639, 3.900000000000000799 ) ) ;
#4753=CARTESIAN_POINT ( 'NONE',  ( 3.756430356250003655, -8.999999999999992895, 2.953124999385485339 ) ) ;
#4781=CARTESIAN_POINT ( 'NONE',  ( 3.999999999999976019, -11.30940107675851536, 0.4124999999999983125 ) ) ;
#4789=CARTESIAN_POINT ( 'NONE',  ( 2.620986760973688460E-15, -13.61880215351699874, 4.331249998770966059 ) ) ;
#4802=MANIFOLD_SOLID_BREP ( 'Cavity1', #11284 ) ;
#4823=DIRECTION ( 'NONE',  ( -0.000000000000000000, -0.000000000000000000, 1.000000000000000000 ) ) ;
#4825=CARTESIAN_POINT ( 'NONE',  ( 1.878215178125004048, -5.746835883940462963, 3.028124999385484184 ) ) ;
#4849=ORIENTED_EDGE ( 'NONE', *, *, #17515, .F. ) ;
#4856=CARTESIAN_POINT ( 'NONE',  ( 1.878215178125004048, -5.746835883940462963, 1.115624999385483207 ) ) ;
#4861=CARTESIAN_POINT ( 'NONE',  ( -3.999999999999996003, -6.690598923241487306, 0.1875000000000008882 ) ) ;
#4862=DIRECTION ( 'NONE',  ( -0.000000000000000000, -0.000000000000000000, -1.000000000000000000 ) ) ;
#4866=CARTESIAN_POINT ( 'NONE',  ( -3.756430356249996994, -8.999999999999992895, 2.278124999385483740 ) ) ;
#4948=CARTESIAN_POINT ( 'NONE',  ( 3.756430356250004099, -6.831223922626973533, 1.190624999385485383 ) ) ;
#4955=UNCERTAINTY_MEASURE_WITH_UNIT (LENGTH_MEASURE( 1.000000000000000082E-05 ), #21934, 'distance_accuracy_value', 'NONE');
#4977=EDGE_LOOP ( 'NONE', ( #8413, #2785, #3317, #23775, #21418, #7446, #23268, #15188, #18106, #13777, #12631, #5526, #9917, #9537, #5487, #11999, #1893, #15334, #14245, #10688, #2276, #25632, #5722 ) ) ;
#4985=CARTESIAN_POINT ( 'NONE',  ( -3.756430356249996994, -8.999999999999992895, 4.528124999385485516 ) ) ;
#4992=CARTESIAN_POINT ( 'NONE',  ( -1.878215178124995832, -5.746835883940462963, 4.340624999385481964 ) ) ;
#4996=LINE ( 'NONE', #13113, #8830 ) ;
#4997=CARTESIAN_POINT ( 'NONE',  ( -3.756430356249997438, -11.16877607737301048, 4.115624999385481431 ) ) ;
#4998=CARTESIAN_POINT ( 'NONE',  ( 3.469446951953614189E-15, -8.999999999999992895, 0.000000000000000000 ) ) ;
#5032=AXIS2_PLACEMENT_3D ( 'NONE', #11971, #2046, #5706 ) ;
#5069=CARTESIAN_POINT ( 'NONE',  ( -1.999999999999998224, -12.46410161513774639, 2.999999999999999112 ) ) ;
#5074=CARTESIAN_POINT ( 'NONE',  ( 4.000000000000003553, -8.999999999999992895, 3.543749998770967302 ) ) ;
#5086=CARTESIAN_POINT ( 'NONE',  ( 2.672651547586948120E-15, -13.33755215474603162, 1.378124999385482274 ) ) ;
#5098=CARTESIAN_POINT ( 'NONE',  ( 3.999999999999976019, -11.30940107675851536, 0.8062499987709651483 ) ) ;
#5125=CARTESIAN_POINT ( 'NONE',  ( -3.756430356249997882, -11.16877607737301226, 1.303124999385484095 ) ) ;
#5126=CARTESIAN_POINT ( 'NONE',  ( 2.000000000000000888, -12.46410161513774817, 1.668749998770965970 ) ) ;
#5130=CARTESIAN_POINT ( 'NONE',  ( 3.735045420075836212E-15, -4.662447845253954171, 4.303124999385482319 ) ) ;
#5136=CARTESIAN_POINT ( 'NONE',  ( -3.756430356249997438, -11.16877607737301048, 3.665624999385481697 ) ) ;
#5140=ORIENTED_EDGE ( 'NONE', *, *, #1839, .F. ) ;
#5178=CARTESIAN_POINT ( 'NONE',  ( 3.469446951953614189E-15, -8.999999999999992895, 18.00000000000000000 ) ) ;
#5183=( GEOMETRIC_REPRESENTATION_CONTEXT ( 3 ) GLOBAL_UNCERTAINTY_ASSIGNED_CONTEXT ( ( #8895 ) ) GLOBAL_UNIT_ASSIGNED_CONTEXT ( ( #19711, #17117, #15166 ) ) REPRESENTATION_CONTEXT ( 'NONE', 'WORKASPACE' ) );
#5199=CARTESIAN_POINT ( 'NONE',  ( 3.469446951953614189E-15, -8.999999999999992895, 0.000000000000000000 ) ) ;
#5207=ORIENTED_EDGE ( 'NONE', *, *, #11447, .T. ) ;
#5213=CARTESIAN_POINT ( 'NONE',  ( -3.756430356249996105, -6.831223922626973533, 1.678124999385481875 ) ) ;
#5214=CARTESIAN_POINT ( 'NONE',  ( 2.672651547586948120E-15, -13.33755215474602984, 3.290624999385483918 ) ) ;
#5215=DIRECTION ( 'NONE',  ( -1.000000000000000000, 0.000000000000000000, 0.000000000000000000 ) ) ;
#5242=CARTESIAN_POINT ( 'NONE',  ( 2.672651547586948120E-15, -13.33755215474602984, 0.9281249993854824298 ) ) ;
#5243=CARTESIAN_POINT ( 'NONE',  ( 2.000000000000000888, -12.46410161513774817, 2.568749998770967213 ) ) ;
#5248=CARTESIAN_POINT ( 'NONE',  ( -1.999999999999995781, -5.535898384862237620, 0.5999999999999998668 ) ) ;
#5252=( BOUNDED_CURVE ( )  B_SPLINE_CURVE ( 2, ( #10255, #10644, #12231, #24641, #22421, #4781, #10769 ),
 .UNSPECIFIED., .F., .F. ) 
 B_SPLINE_CURVE_WITH_KNOTS ( ( 3, 2, 2, 3 ),
 ( 0.04999999999999990563, 0.06666666666666654084, 0.08333333333333316217, 0.09999999999999981126 ),
 .UNSPECIFIED. ) 
 CURVE ( )  GEOMETRIC_REPRESENTATION_ITEM ( )  RATIONAL_B_SPLINE_CURVE ( ( 1.000000000000000666, 0.8660254037844378194, 1.000000000000000000, 0.8660254037844387076, 1.000000000000000000, 0.8660254037844402619, 0.9999999999999984457 ) ) 
 REPRESENTATION_ITEM ( '' )  );
#5259=ORIENTED_EDGE ( 'NONE', *, *, #9136, .F. ) ;
#5262=DIRECTION ( 'NONE',  ( -0.000000000000000000, -0.000000000000000000, -1.000000000000000000 ) ) ;
#5284=LINE ( 'NONE', #11910, #2053 ) ;
#5315=CARTESIAN_POINT ( 'NONE',  ( 4.000000000000032863, -11.30940107675847983, 3.112500000000002487 ) ) ;
#5329=CARTESIAN_POINT ( 'NONE',  ( 3.756430356250003211, -6.831223922626973533, 1.978124999385481919 ) ) ;
#5332=CARTESIAN_POINT ( 'NONE',  ( -3.756430356249996994, -8.999999999999992895, 4.078124999385482674 ) ) ;
#5353=ORIENTED_EDGE ( 'NONE', *, *, #13246, .T. ) ;
#5362=CARTESIAN_POINT ( 'NONE',  ( -1.878215178124998497, -12.25316411605951927, 0.8906249993854836733 ) ) ;
#5363=CARTESIAN_POINT ( 'NONE',  ( -3.999999999999996003, -6.690598923241487306, 2.831249998770966059 ) ) ;
#5369=CARTESIAN_POINT ( 'NONE',  ( -3.999999999999996447, -8.999999999999992895, 1.574999999999999956 ) ) ;
#5376=CARTESIAN_POINT ( 'NONE',  ( 3.756430356250002323, -11.16877607737301403, 3.365624999385485872 ) ) ;
#5383=CARTESIAN_POINT ( 'NONE',  ( 3.469446951953614189E-15, -8.999999999999992895, 18.00000000000000000 ) ) ;
#5385=VERTEX_POINT ( 'NONE', #3056 ) ;
#5432=DIRECTION ( 'NONE',  ( -1.000000000000000000, 0.000000000000000000, 0.000000000000000000 ) ) ;
#5440=CARTESIAN_POINT ( 'NONE',  ( -3.999999999999996447, -8.999999999999992895, 18.00000000000000000 ) ) ;
#5447=DIRECTION ( 'NONE',  ( -0.000000000000000000, -0.000000000000000000, 1.000000000000000000 ) ) ;
#5461=CARTESIAN_POINT ( 'NONE',  ( -1.878215178124995832, -5.746835883940462963, 0.7406249993854828739 ) ) ;
#5463=CARTESIAN_POINT ( 'NONE',  ( 1.878215178125000939, -12.25316411605952283, 3.328124999385485783 ) ) ;
#5487=ORIENTED_EDGE ( 'NONE', *, *, #3339, .F. ) ;
#5498=CARTESIAN_POINT ( 'NONE',  ( -1.878215178124998497, -12.25316411605951927, 3.590624999385481075 ) ) ;
#5499=CARTESIAN_POINT ( 'NONE',  ( -1.999999999999998224, -12.46410161513774639, 1.143749998770968279 ) ) ;
#5506=CARTESIAN_POINT ( 'NONE',  ( 4.000000000000003553, -8.999999999999992895, 2.700000000000001066 ) ) ;
#5526=ORIENTED_EDGE ( 'NONE', *, *, #16679, .F. ) ;
#5528=EDGE_CURVE ( 'NONE', #9327, #17764, #2051, .T. ) ;
#5556=EDGE_CURVE ( 'NONE', #21696, #1445, #16481, .T. ) ;
#5566=EDGE_CURVE ( 'NONE', #20798, #22527, #8189, .T. ) ;
#5590=FACE_OUTER_BOUND ( 'NONE', #19770, .T. ) ;
#5597=CARTESIAN_POINT ( 'NONE',  ( 3.756430356250003211, -6.831223922626973533, 0.1781249993854828739 ) ) ;
#5598=CARTESIAN_POINT ( 'NONE',  ( 1.878215178125000939, -12.25316411605952283, 4.228124999385483918 ) ) ;
#5628=CARTESIAN_POINT ( 'NONE',  ( 1.878215178125004048, -5.746835883940462963, 3.815624999385484273 ) ) ;
#5629=CARTESIAN_POINT ( 'NONE',  ( 2.620986760973688460E-15, -13.61880215351699874, 2.981249998770966414 ) ) ;
#5634=CARTESIAN_POINT ( 'NONE',  ( 2.000000000000000888, -12.46410161513774817, 1.725000000000000755 ) ) ;
#5642=CARTESIAN_POINT ( 'NONE',  ( 4.000000000000001776, -11.30940107675849760, 4.856249998770968190 ) ) ;
#5658=FACE_OUTER_BOUND ( 'NONE', #23123, .T. ) ;
#5662=EDGE_CURVE ( 'NONE', #13093, #6968, #25229, .T. ) ;
#5688=CARTESIAN_POINT ( 'NONE',  ( -4.000000000000039968, -11.30940107675846740, 1.106249998770968634 ) ) ;
#5706=DIRECTION ( 'NONE',  ( -1.000000000000000000, 0.000000000000000000, 0.000000000000000000 ) ) ;
#5711=( BOUNDED_CURVE ( )  B_SPLINE_CURVE ( 2, ( #24376, #4229, #24493, #4091, #22534, #16141, #16532 ),
 .UNSPECIFIED., .F., .T. ) 
 B_SPLINE_CURVE_WITH_KNOTS ( ( 3, 2, 2, 3 ),
 ( 0.3999999999999999667, 0.4166666666666665741, 0.4333333333333332371, 0.4499999999999998446 ),
 .UNSPECIFIED. ) 
 CURVE ( )  GEOMETRIC_REPRESENTATION_ITEM ( )  RATIONAL_B_SPLINE_CURVE ( ( 1.000000000000000444, 0.8660254037844382635, 1.000000000000000000, 0.8660254037844387076, 1.000000000000000000, 0.8660254037844400399, 0.9999999999999986677 ) ) 
 REPRESENTATION_ITEM ( '' )  );
#5712=CARTESIAN_POINT ( 'NONE',  ( 2.672651547586948120E-15, -13.33755215474603162, 2.728124999385481253 ) ) ;
#5720=CARTESIAN_POINT ( 'NONE',  ( 4.000000000000003553, -8.999999999999992895, 2.193749998770967213 ) ) ;
#5722=ORIENTED_EDGE ( 'NONE', *, *, #3893, .F. ) ;
#5731=CARTESIAN_POINT ( 'NONE',  ( -1.999999999999998224, -12.46410161513774639, 2.550000000000000266 ) ) ;
#5734=ORIENTED_EDGE ( 'NONE', *, *, #23260, .T. ) ;
#5744=CARTESIAN_POINT ( 'NONE',  ( 3.735045420075836212E-15, -4.662447845253954171, 2.053124999385483207 ) ) ;
#5745=CARTESIAN_POINT ( 'NONE',  ( 4.000000000000001776, -11.30940107675849760, 4.406249998770963572 ) ) ;
#5749=CARTESIAN_POINT ( 'NONE',  ( 2.000000000000003997, -5.535898384862238508, 2.325000000000000622 ) ) ;
#5751=CARTESIAN_POINT ( 'NONE',  ( -1.999999999999998224, -12.46410161513774639, 2.493749998770968812 ) ) ;
#5757=CARTESIAN_POINT ( 'NONE',  ( -1.999999999999998224, -12.46410161513774639, 1.649999999999998579 ) ) ;
#5784=CARTESIAN_POINT ( 'NONE',  ( -3.756430356249996994, -8.999999999999992895, 0.4781249993854840286 ) ) ;
#5813=CARTESIAN_POINT ( 'NONE',  ( 4.000000000000003553, -6.690598923241489970, 0.03749999999999697325 ) ) ;
#5815=CARTESIAN_POINT ( 'NONE',  ( 2.000000000000000888, -12.46410161513774817, 1.218749998770966902 ) ) ;
#5824=VECTOR ( 'NONE', #12697, 1000.000000000000000 ) ;
#5844=CARTESIAN_POINT ( 'NONE',  ( -1.878215178124998497, -12.25316411605951927, 4.040624999385483918 ) ) ;
#5854=CYLINDRICAL_SURFACE ( 'NONE', #24175, 4.000000000000000000 ) ;
#5870=VECTOR ( 'NONE', #22003, 1000.000000000000000 ) ;
#5882=CARTESIAN_POINT ( 'NONE',  ( -1.878215178124995832, -5.746835883940462963, 1.640624999385484450 ) ) ;
#5883=CARTESIAN_POINT ( 'NONE',  ( 2.620986760973688460E-15, -13.61880215351699874, 3.881249998770965437 ) ) ;
#5888=CARTESIAN_POINT ( 'NONE',  ( -1.999999999999998224, -12.46410161513774639, 1.593749998770967125 ) ) ;
#5889=CARTESIAN_POINT ( 'NONE',  ( 2.620986760973688460E-15, -13.61880215351699874, 1.687500000000000000 ) ) ;
#5913=VECTOR ( 'NONE', #10901, 1000.000000000000000 ) ;
#5916=CARTESIAN_POINT ( 'NONE',  ( 3.735045420075836212E-15, -4.662447845253954171, 0.8156249993854834957 ) ) ;
#5953=CARTESIAN_POINT ( 'NONE',  ( 3.752267015613588906E-15, -4.381197846482986158, 0.1124999999999989203 ) ) ;
#5959=CARTESIAN_POINT ( 'NONE',  ( 2.000000000000003997, -5.535898384862238508, 4.518749998770967835 ) ) ;
#5978=ADVANCED_BREP_SHAPE_REPRESENTATION ( '', ( #4802, #21036 ), #5183 ) ;
#5979=CARTESIAN_POINT ( 'NONE',  ( 3.756430356250003655, -8.999999999999992895, 3.290624999385483029 ) ) ;
#5982=DIRECTION ( 'NONE',  ( -0.000000000000000000, -0.000000000000000000, -1.000000000000000000 ) ) ;
#6013=CARTESIAN_POINT ( 'NONE',  ( -3.756430356249996994, -8.999999999999992895, 2.165624999385482141 ) ) ;
#6014=CARTESIAN_POINT ( 'NONE',  ( 3.752267015613588906E-15, -4.381197846482986158, 4.106249998770966414 ) ) ;
#6033=VERTEX_POINT ( 'NONE', #11948 ) ;
#6037=ORIENTED_EDGE ( 'NONE', *, *, #344, .T. ) ;
#6045=FACE_OUTER_BOUND ( 'NONE', #24408, .T. ) ;
#6048=FACE_OUTER_BOUND ( 'NONE', #12432, .T. ) ;
#6049=PLANE ( 'NONE',  #8799 ) ;
#6087=CARTESIAN_POINT ( 'NONE',  ( -3.999999999999996447, -8.999999999999992895, 18.00000000000000000 ) ) ;
#6100=CARTESIAN_POINT ( 'NONE',  ( -3.756430356249996105, -6.831223922626973533, 2.128124999385481608 ) ) ;
#6103=( NAMED_UNIT ( * ) PLANE_ANGLE_UNIT ( ) SI_UNIT ( $, .RADIAN. ) );
#6118=CARTESIAN_POINT ( 'NONE',  ( -3.999999999999996447, -8.999999999999992895, 2.925000000000000711 ) ) ;
#6119=ORIENTED_EDGE ( 'NONE', *, *, #3875, .F. ) ;
#6123=DIRECTION ( 'NONE',  ( -0.000000000000000000, -0.000000000000000000, -1.000000000000000000 ) ) ;
#6135=CARTESIAN_POINT ( 'NONE',  ( 3.756430356250002323, -11.16877607737301226, 4.153124999385482852 ) ) ;
#6136=CARTESIAN_POINT ( 'NONE',  ( -3.999999999999996003, -6.690598923241487306, 3.281249998770966236 ) ) ;
#6144=LINE ( 'NONE', #6408, #16812 ) ;
#6147=CARTESIAN_POINT ( 'NONE',  ( -3.999999999999996447, -8.999999999999992895, 2.925000000000000711 ) ) ;
#6163=EDGE_CURVE ( 'NONE', #11292, #523, #24385, .T. ) ;
#6164=CARTESIAN_POINT ( 'NONE',  ( 1.878215178125004048, -5.746835883940462963, 2.578124999385485339 ) ) ;
#6171=CARTESIAN_POINT ( 'NONE',  ( -3.756430356249996994, -8.999999999999992895, 1.715624999385483074 ) ) ;
#6174=CARTESIAN_POINT ( 'NONE',  ( 3.999999999999987121, -11.30940107675850648, 3.562499999999996891 ) ) ;
#6199=CARTESIAN_POINT ( 'NONE',  ( 4.000000000000003553, -8.999999999999992895, 1.293749998770969079 ) ) ;
#6202=CARTESIAN_POINT ( 'NONE',  ( -1.999999999999998224, -12.46410161513774639, 2.100000000000000977 ) ) ;
#6224=CARTESIAN_POINT ( 'NONE',  ( 3.756430356250003211, -6.831223922626973533, 2.878124999385481608 ) ) ;
#6234=CARTESIAN_POINT ( 'NONE',  ( 3.469446951953614189E-15, -8.999999999999992895, 18.00000000000000000 ) ) ;
#6267=CARTESIAN_POINT ( 'NONE',  ( -3.999999999999996447, -8.999999999999992895, 4.218749998770966236 ) ) ;
#6280=CARTESIAN_POINT ( 'NONE',  ( 3.469446951953614189E-15, -8.999999999999992895, 18.00000000000000000 ) ) ;
#6301=CARTESIAN_POINT ( 'NONE',  ( -1.878215178124995832, -5.746835883940462963, 1.753124999385485827 ) ) ;
#6302=CARTESIAN_POINT ( 'NONE',  ( 3.999999999999954259, -6.690598923241460660, 1.331249998770968057 ) ) ;
#6307=CARTESIAN_POINT ( 'NONE',  ( 1.878215178125000939, -12.25316411605952283, 1.415624999385481253 ) ) ;
#6311=CARTESIAN_POINT ( 'NONE',  ( 3.735045420075836212E-15, -4.662447845253954171, 1.715624999385482852 ) ) ;
#6346=CARTESIAN_POINT ( 'NONE',  ( -1.999999999999995781, -5.535898384862237620, 1.500000000000001332 ) ) ;
#6367=CARTESIAN_POINT ( 'NONE',  ( -4.000000000000033751, -6.690598923241509510, 1.087499999999997025 ) ) ;
#6368=SURFACE_STYLE_FILL_AREA ( #11979 ) ;
#6370=CARTESIAN_POINT ( 'NONE',  ( -3.999999999999996447, -8.999999999999992895, 3.374999999999999556 ) ) ;
#6398=CARTESIAN_POINT ( 'NONE',  ( 3.735045420075836212E-15, -4.662447845253954171, 4.303124999385482319 ) ) ;
#6399=CARTESIAN_POINT ( 'NONE',  ( -3.756430356249995661, -6.831223922626973533, 3.140624999385484006 ) ) ;
#6403=CARTESIAN_POINT ( 'NONE',  ( 4.000000000000051514, -11.30940107675846917, 0.8624999999999993783 ) ) ;
#6408=CARTESIAN_POINT ( 'NONE',  ( -3.999999999999996447, -8.999999999999992895, 18.00000000000000000 ) ) ;
#6410=CARTESIAN_POINT ( 'NONE',  ( 4.000000000000003553, -8.999999999999992895, 2.193749998770967213 ) ) ;
#6428=ORIENTED_EDGE ( 'NONE', *, *, #19749, .F. ) ;
#6430=DIRECTION ( 'NONE',  ( 1.000000000000000000, 0.000000000000000000, 0.000000000000000000 ) ) ;
#6432=CARTESIAN_POINT ( 'NONE',  ( -3.756430356249996994, -8.999999999999992895, 3.628124999385483829 ) ) ;
#6438=CARTESIAN_POINT ( 'NONE',  ( 3.756430356250004099, -6.831223922626973533, 1.528124999385482186 ) ) ;
#6442=CARTESIAN_POINT ( 'NONE',  ( 3.735045420075836212E-15, -4.662447845253954171, 3.065624999385482052 ) ) ;
#6444=CYLINDRICAL_SURFACE ( 'NONE', #14132, 4.000000000000000000 ) ;
#6507=DIRECTION ( 'NONE',  ( -0.000000000000000000, -0.000000000000000000, -1.000000000000000000 ) ) ;
#6519=CARTESIAN_POINT ( 'NONE',  ( 4.000000000000012434, -6.690598923241494411, 1.837499999999995914 ) ) ;
#6521=CARTESIAN_POINT ( 'NONE',  ( 2.672651547586948120E-15, -13.33755215474602984, 1.040624999385485472 ) ) ;
#6535=ADVANCED_FACE ( 'NONE', ( #5658 ), #21489, .T. ) ;
#6552=CARTESIAN_POINT ( 'NONE',  ( 1.878215178125000939, -12.25316411605952283, 2.878124999385483385 ) ) ;
#6555=LINE ( 'NONE', #6684, #25090 ) ;
#6556=ADVANCED_FACE ( 'NONE', ( #6045 ), #15124, .T. ) ;
#6559=CARTESIAN_POINT ( 'NONE',  ( 3.756430356250002323, -11.16877607737301226, 2.803124999385479210 ) ) ;
#6560=CARTESIAN_POINT ( 'NONE',  ( -3.999999999999996447, -8.999999999999992895, 0.2249999999999995060 ) ) ;
#6561=CARTESIAN_POINT ( 'NONE',  ( 2.000000000000000888, -12.46410161513774817, 3.974999999999999201 ) ) ;
#6564=CARTESIAN_POINT ( 'NONE',  ( 2.672651547586948120E-15, -13.33755215474603162, 2.390624999385484450 ) ) ;
#6566=CARTESIAN_POINT ( 'NONE',  ( 3.469446951953614189E-15, -8.999999999999992895, 18.00000000000000000 ) ) ;
#6567=ORIENTED_EDGE ( 'NONE', *, *, #18928, .T. ) ;
#6608=CARTESIAN_POINT ( 'NONE',  ( 3.756430356250002323, -11.16877607737301403, 4.603124999385482141 ) ) ;
#6611=CARTESIAN_POINT ( 'NONE',  ( 3.752267015613588906E-15, -4.381197846482986158, 3.262500000000001066 ) ) ;
#6622=FACE_OUTER_BOUND ( 'NONE', #19495, .T. ) ;
#6627=CYLINDRICAL_SURFACE ( 'NONE', #3757, 4.000000000000000000 ) ;
#6635=DIRECTION ( 'NONE',  ( -1.000000000000000000, 0.000000000000000000, 0.000000000000000000 ) ) ;
#6645=AXIS2_PLACEMENT_3D ( 'NONE', #10080, #24549, #6635 ) ;
#6648=CARTESIAN_POINT ( 'NONE',  ( -3.999999999999996447, -8.999999999999992895, 3.318749998770968102 ) ) ;
#6649=CARTESIAN_POINT ( 'NONE',  ( -1.878215178124998497, -12.25316411605951927, 1.903124999385483296 ) ) ;
#6667=CARTESIAN_POINT ( 'NONE',  ( 4.000000000000003553, -8.999999999999992895, 3.543749998770967302 ) ) ;
#6676=VERTEX_POINT ( 'NONE', #21533 ) ;
#6681=CARTESIAN_POINT ( 'NONE',  ( -3.756430356249996994, -8.999999999999992895, 1.828124999385484450 ) ) ;
#6684=CARTESIAN_POINT ( 'NONE',  ( -3.999999999999996447, -8.999999999999992895, 18.00000000000000000 ) ) ;
#6686=CARTESIAN_POINT ( 'NONE',  ( 1.878215178125000939, -12.25316411605952283, 2.315624999385482941 ) ) ;
#6688=CARTESIAN_POINT ( 'NONE',  ( 3.752267015613588906E-15, -4.381197846482986158, 3.262500000000001066 ) ) ;
#6692=CARTESIAN_POINT ( 'NONE',  ( 3.756430356250002323, -11.16877607737301403, 2.465624999385482852 ) ) ;
#6702=ORIENTED_EDGE ( 'NONE', *, *, #20767, .F. ) ;
#6737=ORIENTED_EDGE ( 'NONE', *, *, #23613, .F. ) ;
#6788=CARTESIAN_POINT ( 'NONE',  ( -3.756430356249996994, -8.999999999999992895, 1.828124999385484450 ) ) ;
#6794=CARTESIAN_POINT ( 'NONE',  ( 2.000000000000003997, -5.535898384862238508, 1.818749998770966769 ) ) ;
#6805=DIRECTION ( 'NONE',  ( 1.000000000000000000, 0.000000000000000000, 0.000000000000000000 ) ) ;
#6823=CARTESIAN_POINT ( 'NONE',  ( -3.756430356249997882, -11.16877607737301226, 0.8531249993854844726 ) ) ;
#6829=CARTESIAN_POINT ( 'NONE',  ( 1.878215178125000939, -12.25316411605952283, 3.665624999385483473 ) ) ;
#6831=CARTESIAN_POINT ( 'NONE',  ( -3.999999999999996003, -6.690598923241487306, 3.787499999999998757 ) ) ;
#6834=CARTESIAN_POINT ( 'NONE',  ( -1.878215178124998497, -12.25316411605951927, 2.353124999385485694 ) ) ;
#6856=MECHANICAL_DESIGN_GEOMETRIC_PRESENTATION_REPRESENTATION('',(#15619),#24816);
#6874=EDGE_LOOP ( 'NONE', ( #25657, #669 ) ) ;
#6881=CARTESIAN_POINT ( 'NONE',  ( 4.000000000000003553, -8.999999999999992895, 3.149999999999999911 ) ) ;
#6911=CARTESIAN_POINT ( 'NONE',  ( 3.756430356250003655, -8.999999999999992895, 2.953124999385485339 ) ) ;
#6922=CARTESIAN_POINT ( 'NONE',  ( 4.000000000000003553, -8.999999999999992895, 0.8437499987709664584 ) ) ;
#6946=LINE ( 'NONE', #8920, #21956 ) ;
#6948=CARTESIAN_POINT ( 'NONE',  ( 3.735045420075836212E-15, -4.662447845253954171, 0.2531249993854848279 ) ) ;
#6952=CARTESIAN_POINT ( 'NONE',  ( 2.000000000000003997, -5.535898384862238508, 0.5250000000000011324 ) ) ;
#6953=CARTESIAN_POINT ( 'NONE',  ( 3.756430356250004099, -6.831223922626973533, 4.228124999385484806 ) ) ;
#6955=CARTESIAN_POINT ( 'NONE',  ( -3.999999999999996447, -8.999999999999992895, 3.374999999999999556 ) ) ;
#6958=CARTESIAN_POINT ( 'NONE',  ( -1.878215178124995832, -5.746835883940462963, 4.003124999385484273 ) ) ;
#6968=VERTEX_POINT ( 'NONE', #586 ) ;
#6977=CARTESIAN_POINT ( 'NONE',  ( 3.469446951953614189E-15, -8.999999999999992895, 18.00000000000000000 ) ) ;
#7007=AXIS2_PLACEMENT_3D ( 'NONE', #4998, #20961, #11397 ) ;
#7036=CARTESIAN_POINT ( 'NONE',  ( 3.756430356250003655, -8.999999999999992895, 4.303124999385482319 ) ) ;
#7050=CARTESIAN_POINT ( 'NONE',  ( 3.878215178125003604, -8.999999999999992895, 0.3234374990782259984 ) ) ;
#7061=ORIENTED_EDGE ( 'NONE', *, *, #19431, .F. ) ;
#7066=CARTESIAN_POINT ( 'NONE',  ( 3.469446951953614189E-15, -8.999999999999992895, 18.00000000000000000 ) ) ;
#7071=CARTESIAN_POINT ( 'NONE',  ( 3.756430356250003655, -8.999999999999992895, 1.040624999385484584 ) ) ;
#7079=CARTESIAN_POINT ( 'NONE',  ( -3.756430356249997882, -11.16877607737301226, 4.003124999385478056 ) ) ;
#7086=CARTESIAN_POINT ( 'NONE',  ( 1.878215178125000939, -12.25316411605952283, 4.678124999385483207 ) ) ;
#7177=CARTESIAN_POINT ( 'NONE',  ( 3.756430356250002323, -11.16877607737301226, 3.365624999385485872 ) ) ;
#7210=CARTESIAN_POINT ( 'NONE',  ( -3.756430356249995661, -6.831223922626973533, 0.3281249993854827851 ) ) ;
#7211=CARTESIAN_POINT ( 'NONE',  ( 2.620986760973688460E-15, -13.61880215351699874, 1.631249998770966991 ) ) ;
#7216=CARTESIAN_POINT ( 'NONE',  ( -3.756430356249997882, -11.16877607737301226, 3.553124999385482763 ) ) ;
#7221=CARTESIAN_POINT ( 'NONE',  ( 3.752267015613588906E-15, -4.381197846482986158, 0.5062499987709696558 ) ) ;
#7286=PRODUCT_DEFINITION_FORMATION_WITH_SPECIFIED_SOURCE ( 'ANY', '', #12142, .NOT_KNOWN. ) ;
#7304=CARTESIAN_POINT ( 'NONE',  ( 3.756430356250003655, -8.999999999999992895, 1.490624999385483429 ) ) ;
#7305=CARTESIAN_POINT ( 'NONE',  ( 3.756430356250003655, -8.999999999999992895, 3.853124999385483473 ) ) ;
#7332=CARTESIAN_POINT ( 'NONE',  ( 3.735045420075836212E-15, -4.662447845253954171, 3.965624999385486404 ) ) ;
#7333=CARTESIAN_POINT ( 'NONE',  ( -1.999999999999998224, -12.46410161513774639, 2.043749998770966414 ) ) ;
#7339=CARTESIAN_POINT ( 'NONE',  ( 2.672651547586948120E-15, -13.33755215474602984, 3.628124999385485161 ) ) ;
#7345=CARTESIAN_POINT ( 'NONE',  ( 2.672651547586948120E-15, -13.33755215474603162, 3.740624999385483651 ) ) ;
#7351=VERTEX_POINT ( 'NONE', #16252 ) ;
#7367=FACE_OUTER_BOUND ( 'NONE', #14655, .T. ) ;
#7390=( BOUNDED_CURVE ( )  B_SPLINE_CURVE ( 2, ( #2693, #14731, #22708, #4789, #12764, #860, #2813 ),
 .UNSPECIFIED., .F., .F. ) 
 B_SPLINE_CURVE_WITH_KNOTS ( ( 3, 2, 2, 3 ),
 ( 0.8499999999999998668, 0.8666666666666664742, 0.8833333333333330817, 0.8999999999999996891 ),
 .UNSPECIFIED. ) 
 CURVE ( )  GEOMETRIC_REPRESENTATION_ITEM ( )  RATIONAL_B_SPLINE_CURVE ( ( 1.000000000000000888, 0.8660254037844378194, 1.000000000000000000, 0.8660254037844387076, 1.000000000000000000, 0.8660254037844413721, 0.9999999999999973355 ) ) 
 REPRESENTATION_ITEM ( '' )  );
#7418=CARTESIAN_POINT ( 'NONE',  ( 3.756430356250002323, -11.16877607737301403, 0.5531249993854806535 ) ) ;
#7420=CARTESIAN_POINT ( 'NONE',  ( -3.756430356249997882, -11.16877607737301226, 4.565624999385485161 ) ) ;
#7446=ORIENTED_EDGE ( 'NONE', *, *, #344, .F. ) ;
#7453=CARTESIAN_POINT ( 'NONE',  ( -3.756430356249996994, -8.999999999999992895, 3.515624999385482674 ) ) ;
#7454=CARTESIAN_POINT ( 'NONE',  ( 4.000000000000001776, -11.30940107675849760, 2.156249998770968457 ) ) ;
#7458=CARTESIAN_POINT ( 'NONE',  ( -3.999999999999996447, -8.999999999999992895, 18.00000000000000000 ) ) ;
#7459=CARTESIAN_POINT ( 'NONE',  ( 4.000000000000003553, -6.690598923241489970, 0.9375000000000004441 ) ) ;
#7465=CARTESIAN_POINT ( 'NONE',  ( -1.878215178124995832, -5.746835883940462963, 3.553124999385485427 ) ) ;
#7487=CARTESIAN_POINT ( 'NONE',  ( 3.756430356250003655, -8.999999999999992895, 0.7031249993854835623 ) ) ;
#7533=VERTEX_POINT ( 'NONE', #13363 ) ;
#7550=CARTESIAN_POINT ( 'NONE',  ( 3.756430356250003211, -6.831223922626973533, 1.078124999385482230 ) ) ;
#7554=CARTESIAN_POINT ( 'NONE',  ( 1.878215178125004048, -5.746835883940462963, 3.478124999385483029 ) ) ;
#7571=CARTESIAN_POINT ( 'NONE',  ( 4.000000000000001776, -11.30940107675849760, 4.462500000000000355 ) ) ;
#7592=CARTESIAN_POINT ( 'NONE',  ( 1.878215178125000939, -12.25316411605952283, 3.215624999385484184 ) ) ;
#7593=CARTESIAN_POINT ( 'NONE',  ( -1.999999999999998224, -12.46410161513774639, 2.943749998770967657 ) ) ;
#7599=CARTESIAN_POINT ( 'NONE',  ( -3.999999999999996447, -8.999999999999992895, 2.474999999999997868 ) ) ;
#7624=CARTESIAN_POINT ( 'NONE',  ( 3.735045420075836212E-15, -4.662447845253954171, 1.265624999385483118 ) ) ;
#7629=( GEOMETRIC_REPRESENTATION_CONTEXT ( 3 ) GLOBAL_UNCERTAINTY_ASSIGNED_CONTEXT ( ( #24841 ) ) GLOBAL_UNIT_ASSIGNED_CONTEXT ( ( #15539, #8073, #17622 ) ) REPRESENTATION_CONTEXT ( 'NONE', 'WORKASPACE' ) );
#7666=DIRECTION ( 'NONE',  ( -0.000000000000000000, -0.000000000000000000, -1.000000000000000000 ) ) ;
#7683=CARTESIAN_POINT ( 'NONE',  ( 2.672651547586948120E-15, -13.33755215474603162, 4.078124999385480010 ) ) ;
#7710=ORIENTED_EDGE ( 'NONE', *, *, #11535, .F. ) ;
#7718=CARTESIAN_POINT ( 'NONE',  ( -3.756430356249997882, -11.16877607737301226, 4.003124999385478056 ) ) ;
#7719=CARTESIAN_POINT ( 'NONE',  ( 3.752267015613588906E-15, -4.381197846482986158, 4.556249998770967480 ) ) ;
#7724=CARTESIAN_POINT ( 'NONE',  ( 4.000000000000003553, -6.690598923241489970, 2.287499999999995648 ) ) ;
#7731=CARTESIAN_POINT ( 'NONE',  ( 3.752267015613588906E-15, -4.381197846482986158, 3.206249998770963838 ) ) ;
#7755=CARTESIAN_POINT ( 'NONE',  ( 4.000000000000003553, -8.999999999999992895, 18.00000000000000000 ) ) ;
#7795=VERTEX_POINT ( 'NONE', #8242 ) ;
#7804=EDGE_CURVE ( 'NONE', #10048, #702, #17788, .T. ) ;
#7805=CARTESIAN_POINT ( 'NONE',  ( -3.756430356249996994, -8.999999999999992895, 2.165624999385482141 ) ) ;
#7809=CARTESIAN_POINT ( 'NONE',  ( -3.999999999999996447, -8.999999999999992895, 3.824999999999998401 ) ) ;
#7826=ORIENTED_EDGE ( 'NONE', *, *, #8861, .T. ) ;
#7837=CARTESIAN_POINT ( 'NONE',  ( 3.756430356250004099, -6.831223922626973533, 1.978124999385481697 ) ) ;
#7838=CARTESIAN_POINT ( 'NONE',  ( 2.000000000000003997, -5.535898384862238508, 3.618749998770966148 ) ) ;
#7843=CARTESIAN_POINT ( 'NONE',  ( -1.999999999999995781, -5.535898384862237620, 2.849999999999998312 ) ) ;
#7858=VECTOR ( 'NONE', #11008, 1000.000000000000000 ) ;
#7869=CARTESIAN_POINT ( 'NONE',  ( 1.878215178125000939, -12.25316411605952283, 0.6281249993854848279 ) ) ;
#7878=CARTESIAN_POINT ( 'NONE',  ( -3.999999999999997335, -11.30940107675849404, 3.412499999999996980 ) ) ;
#7902=EDGE_CURVE ( 'NONE', #17175, #10674, #6144, .T. ) ;
#7906=CARTESIAN_POINT ( 'NONE',  ( 2.000000000000003997, -5.535898384862238508, 0.07499999999999867883 ) ) ;
#7914=( BOUNDED_CURVE ( )  B_SPLINE_CURVE ( 2, ( #19892, #6302, #15998, #2380, #294, #429, #24353 ),
 .UNSPECIFIED., .F., .F. ) 
 B_SPLINE_CURVE_WITH_KNOTS ( ( 3, 2, 2, 3 ),
 ( 0.2000000000000003719, 0.2166666666666670071, 0.2333333333333336423, 0.2500000000000002776 ),
 .UNSPECIFIED. ) 
 CURVE ( )  GEOMETRIC_REPRESENTATION_ITEM ( )  RATIONAL_B_SPLINE_CURVE ( ( 0.9999999999999971134, 0.8660254037844415942, 1.000000000000000000, 0.8660254037844387076, 1.000000000000000000, 0.8660254037844364872, 1.000000000000002220 ) ) 
 REPRESENTATION_ITEM ( '' )  );
#7925=( BOUNDED_CURVE ( )  B_SPLINE_CURVE ( 2, ( #6667, #12168, #18317, #12698, #10591, #668, #10322 ),
 .UNSPECIFIED., .F., .F. ) 
 B_SPLINE_CURVE_WITH_KNOTS ( ( 3, 2, 2, 3 ),
 ( 0.7000000000000001776, 0.7166666666666667851, 0.7333333333333333925, 0.7500000000000000000 ),
 .UNSPECIFIED. ) 
 CURVE ( )  GEOMETRIC_REPRESENTATION_ITEM ( )  RATIONAL_B_SPLINE_CURVE ( ( 0.9999999999999982236, 0.8660254037844404840, 1.000000000000000000, 0.8660254037844387076, 1.000000000000000000, 0.8660254037844387076, 1.000000000000000000 ) ) 
 REPRESENTATION_ITEM ( '' )  );
#7936=CARTESIAN_POINT ( 'NONE',  ( -1.878215178124998497, -12.25316411605951927, 2.240624999385484095 ) ) ;
#7937=EDGE_CURVE ( 'NONE', #337, #10048, #2887, .T. ) ;
#7946=DIRECTION ( 'NONE',  ( -1.000000000000000000, 0.000000000000000000, 0.000000000000000000 ) ) ;
#7955=EDGE_CURVE ( 'NONE', #13093, #9331, #13078, .T. ) ;
#7965=ORIENTED_EDGE ( 'NONE', *, *, #5662, .F. ) ;
#7970=AXIS2_PLACEMENT_3D ( 'NONE', #776, #22627, #12938 ) ;
#7977=CARTESIAN_POINT ( 'NONE',  ( -3.756430356249996994, -8.999999999999992895, 3.065624999385483385 ) ) ;
#7978=CARTESIAN_POINT ( 'NONE',  ( 2.000000000000003997, -5.535898384862238508, 4.068749998770968546 ) ) ;
#7983=CARTESIAN_POINT ( 'NONE',  ( 2.000000000000000888, -12.46410161513774817, 0.8249999999999992895 ) ) ;
#8012=CARTESIAN_POINT ( 'NONE',  ( 3.756430356250002323, -11.16877607737301226, 1.115624999385483429 ) ) ;
#8017=FACE_BOUND ( 'NONE', #22744, .T. ) ;
#8051=CARTESIAN_POINT ( 'NONE',  ( 4.000000000000003553, -8.999999999999992895, 2.700000000000001066 ) ) ;
#8073=( NAMED_UNIT ( * ) PLANE_ANGLE_UNIT ( ) SI_UNIT ( $, .RADIAN. ) );
#8076=CARTESIAN_POINT ( 'NONE',  ( 1.878215178125004048, -5.746835883940462963, 2.465624999385483740 ) ) ;
#8090=( BOUNDED_CURVE ( )  B_SPLINE_CURVE ( 2, ( #6118, #14102, #5069, #25209, #18797, #5315, #19310 ),
 .UNSPECIFIED., .F., .F. ) 
 B_SPLINE_CURVE_WITH_KNOTS ( ( 3, 2, 2, 3 ),
 ( 0.6500000000000002442, 0.6666666666666668517, 0.6833333333333335702, 0.7000000000000001776 ),
 .UNSPECIFIED. ) 
 CURVE ( )  GEOMETRIC_REPRESENTATION_ITEM ( )  RATIONAL_B_SPLINE_CURVE ( ( 0.9999999999999982236, 0.8660254037844404840, 1.000000000000000000, 0.8660254037844387076, 1.000000000000000000, 0.8660254037844369313, 1.000000000000001776 ) ) 
 REPRESENTATION_ITEM ( '' )  );
#8114=CARTESIAN_POINT ( 'NONE',  ( 1.878215178125004048, -5.746835883940462963, 4.265624999385483562 ) ) ;
#8115=CARTESIAN_POINT ( 'NONE',  ( 3.735045420075836212E-15, -4.662447845253954171, 0.3656249993854837066 ) ) ;
#8134=ORIENTED_EDGE ( 'NONE', *, *, #7937, .T. ) ;
#8142=CARTESIAN_POINT ( 'NONE',  ( 3.756430356250003655, -8.999999999999992895, 2.953124999385485339 ) ) ;
#8147=CARTESIAN_POINT ( 'NONE',  ( 3.735045420075836212E-15, -4.662447845253954171, 1.603124999385479921 ) ) ;
#8150=CARTESIAN_POINT ( 'NONE',  ( -3.999999999999996447, -8.999999999999992895, 3.374999999999999556 ) ) ;
#8189=( BOUNDED_CURVE ( )  B_SPLINE_CURVE ( 2, ( #12801, #6519, #20775, #4431, #526, #2853, #10820 ),
 .UNSPECIFIED., .F., .F. ) 
 B_SPLINE_CURVE_WITH_KNOTS ( ( 3, 2, 2, 3 ),
 ( 0.3999999999999999667, 0.4166666666666665741, 0.4333333333333332371, 0.4499999999999998446 ),
 .UNSPECIFIED. ) 
 CURVE ( )  GEOMETRIC_REPRESENTATION_ITEM ( )  RATIONAL_B_SPLINE_CURVE ( ( 1.000000000000000444, 0.8660254037844382635, 1.000000000000000000, 0.8660254037844387076, 1.000000000000000000, 0.8660254037844400399, 0.9999999999999986677 ) ) 
 REPRESENTATION_ITEM ( '' )  );
#8198=CARTESIAN_POINT ( 'NONE',  ( 1.878215178125000939, -12.25316411605952283, 2.315624999385482941 ) ) ;
#8201=( NAMED_UNIT ( * ) SI_UNIT ( $, .STERADIAN. ) SOLID_ANGLE_UNIT ( ) );
#8205=FACE_OUTER_BOUND ( 'NONE', #25006, .T. ) ;
#8232=CARTESIAN_POINT ( 'NONE',  ( -1.878215178124998497, -12.25316411605951927, 0.5531249993854860936 ) ) ;
#8238=CARTESIAN_POINT ( 'NONE',  ( 2.620986760973688460E-15, -13.61880215351699874, 1.631249998770966991 ) ) ;
#8242=CARTESIAN_POINT ( 'NONE',  ( -3.999999999999996447, -8.999999999999992895, 3.824999999999998401 ) ) ;
#8263=CARTESIAN_POINT ( 'NONE',  ( -3.756430356249997882, -11.16877607737301226, 2.765624999385486227 ) ) ;
#8268=AXIS2_PLACEMENT_3D ( 'NONE', #2655, #4473, #16641 ) ;
#8269=CARTESIAN_POINT ( 'NONE',  ( -1.878215178124995832, -5.746835883940462963, 1.190624999385481830 ) ) ;
#8271=DIRECTION ( 'NONE',  ( -0.8660254037844397068, 0.000000000000000000, 0.4999999999999983347 ) ) ;
#8272=CARTESIAN_POINT ( 'NONE',  ( -1.878215178124995832, -5.746835883940462963, 1.303124999385483429 ) ) ;
#8282=ORIENTED_EDGE ( 'NONE', *, *, #10638, .F. ) ;
#8301=CARTESIAN_POINT ( 'NONE',  ( -1.999999999999995781, -5.535898384862237620, 4.593749998770966236 ) ) ;
#8325=CARTESIAN_POINT ( 'NONE',  ( 4.000000000000003553, -8.999999999999992895, 4.049999999999998046 ) ) ;
#8331=DIRECTION ( 'NONE',  ( -0.000000000000000000, -0.000000000000000000, -1.000000000000000000 ) ) ;
#8348=ORIENTED_EDGE ( 'NONE', *, *, #15959, .F. ) ;
#8361=CARTESIAN_POINT ( 'NONE',  ( 1.878215178125004048, -5.746835883940462963, 2.578124999385485339 ) ) ;
#8365=CARTESIAN_POINT ( 'NONE',  ( -3.999999999999996447, -8.999999999999992895, 0.6749999999999984901 ) ) ;
#8388=CARTESIAN_POINT ( 'NONE',  ( -1.999999999999995781, -5.535898384862237620, 2.793749998770966858 ) ) ;
#8390=EDGE_CURVE ( 'NONE', #15232, #1313, #22293, .T. ) ;
#8392=CYLINDRICAL_SURFACE ( 'NONE', #19424, 3.000000000000000444 ) ;
#8396=CARTESIAN_POINT ( 'NONE',  ( 3.735045420075836212E-15, -4.662447845253954171, 2.165624999385483029 ) ) ;
#8403=FACE_OUTER_BOUND ( 'NONE', #18704, .T. ) ;
#8404=CARTESIAN_POINT ( 'NONE',  ( -3.756430356249996994, -8.999999999999992895, 2.615624999385480987 ) ) ;
#8405=CARTESIAN_POINT ( 'NONE',  ( 2.000000000000000888, -12.46410161513774817, 4.424999999999998046 ) ) ;
#8409=CARTESIAN_POINT ( 'NONE',  ( 1.878215178125004048, -5.746835883940462963, 1.228124999385484584 ) ) ;
#8413=ORIENTED_EDGE ( 'NONE', *, *, #1839, .T. ) ;
#8500=CARTESIAN_POINT ( 'NONE',  ( -3.756430356249996994, -8.999999999999992895, 1.378124999385485605 ) ) ;
#8532=CARTESIAN_POINT ( 'NONE',  ( 3.756430356250004099, -6.831223922626973533, 2.090624999385480631 ) ) ;
#8533=CARTESIAN_POINT ( 'NONE',  ( -3.999999999999996447, -8.999999999999992895, 0.6187499987709670357 ) ) ;
#8538=CARTESIAN_POINT ( 'NONE',  ( -3.756430356249997882, -11.16877607737301226, 2.653124999385483296 ) ) ;
#8539=CARTESIAN_POINT ( 'NONE',  ( 4.000000000000001776, -11.30940107675849760, 3.112500000000001155 ) ) ;
#8543=CARTESIAN_POINT ( 'NONE',  ( 2.672651547586948120E-15, -13.33755215474603162, 1.490624999385481209 ) ) ;
#8572=CARTESIAN_POINT ( 'NONE',  ( 3.999999999999972466, -6.690598923241471319, 1.387500000000000844 ) ) ;
#8601=CARTESIAN_POINT ( 'NONE',  ( 3.469446951953614189E-15, -8.999999999999992895, 18.00000000000000000 ) ) ;
#8609=CARTESIAN_POINT ( 'NONE',  ( 4.000000000000003553, -8.999999999999992895, 1.799999999999999600 ) ) ;
#8611=ORIENTED_EDGE ( 'NONE', *, *, #16875, .T. ) ;
#8613=ORIENTED_EDGE ( 'NONE', *, *, #18847, .T. ) ;
#8620=CARTESIAN_POINT ( 'NONE',  ( 2.672651547586948120E-15, -13.33755215474602984, 1.940624999385484717 ) ) ;
#8649=CARTESIAN_POINT ( 'NONE',  ( -3.756430356249997882, -11.16877607737301226, 3.665624999385481697 ) ) ;
#8653=CARTESIAN_POINT ( 'NONE',  ( -3.756430356249996994, -8.999999999999992895, 0.8156249993854814972 ) ) ;
#8655=CARTESIAN_POINT ( 'NONE',  ( -3.999999999999996447, -8.999999999999992895, 3.824999999999998401 ) ) ;
#8658=CARTESIAN_POINT ( 'NONE',  ( -1.878215178124998497, -12.25316411605951927, 2.803124999385484539 ) ) ;
#8683=CARTESIAN_POINT ( 'NONE',  ( 3.999999999999970690, -11.30940107675851536, 2.212499999999996803 ) ) ;
#8742=CARTESIAN_POINT ( 'NONE',  ( -3.756430356249997882, -11.16877607737301226, 2.765624999385486227 ) ) ;
#8753=CARTESIAN_POINT ( 'NONE',  ( 2.000000000000000888, -12.46410161513774817, 0.7687499987709678351 ) ) ;
#8780=CARTESIAN_POINT ( 'NONE',  ( 3.756430356250004099, -6.831223922626973533, 3.890624999385483562 ) ) ;
#8781=FACE_OUTER_BOUND ( 'NONE', #4977, .T. ) ;
#8787=CARTESIAN_POINT ( 'NONE',  ( -3.756430356249997882, -11.16877607737301226, 3.103124999385483029 ) ) ;
#8792=CARTESIAN_POINT ( 'NONE',  ( 1.878215178125000939, -12.25316411605952283, 1.978124999385485250 ) ) ;
#8799=AXIS2_PLACEMENT_3D ( 'NONE', #10218, #18216, #14300 ) ;
#8814=CARTESIAN_POINT ( 'NONE',  ( -3.999999999999996447, -8.999999999999992895, 18.00000000000000000 ) ) ;
#8830=VECTOR ( 'NONE', #1074, 1000.000000000000000 ) ;
#8850=CARTESIAN_POINT ( 'NONE',  ( 3.756430356250003655, -8.999999999999992895, 4.190624999385480720 ) ) ;
#8861=EDGE_CURVE ( 'NONE', #19775, #1445, #23930, .T. ) ;
#8887=CARTESIAN_POINT ( 'NONE',  ( -1.878215178124995832, -5.746835883940462963, 0.8531249993854843616 ) ) ;
#8895=UNCERTAINTY_MEASURE_WITH_UNIT (LENGTH_MEASURE( 1.000000000000000082E-05 ), #19711, 'distance_accuracy_value', 'NONE');
#8899=CARTESIAN_POINT ( 'NONE',  ( 2.620986760973688460E-15, -13.61880215351699874, 0.7312499987709675242 ) ) ;
#8920=CARTESIAN_POINT ( 'NONE',  ( 4.000000000000003553, -8.999999999999992895, 18.00000000000000000 ) ) ;
#8923=CARTESIAN_POINT ( 'NONE',  ( -3.756430356249997882, -11.16877607737301226, 0.4031249993854806868 ) ) ;
#8927=VECTOR ( 'NONE', #4823, 1000.000000000000000 ) ;
#8929=CARTESIAN_POINT ( 'NONE',  ( 4.000000000000003553, -8.999999999999992895, 0.000000000000000000 ) ) ;
#8951=ORIENTED_EDGE ( 'NONE', *, *, #15959, .T. ) ;
#9005=EDGE_CURVE ( 'NONE', #13593, #16478, #1904, .T. ) ;
#9030=VERTEX_POINT ( 'NONE', #24298 ) ;
#9038=CARTESIAN_POINT ( 'NONE',  ( 3.756430356250002323, -11.16877607737301226, 1.003124999385480276 ) ) ;
#9044=CARTESIAN_POINT ( 'NONE',  ( -3.756430356249995661, -6.831223922626973533, 3.928124999385480542 ) ) ;
#9049=CARTESIAN_POINT ( 'NONE',  ( 1.878215178125000939, -12.25316411605952283, 3.778124999385484628 ) ) ;
#9052=ORIENTED_EDGE ( 'NONE', *, *, #6163, .T. ) ;
#9081=CARTESIAN_POINT ( 'NONE',  ( -1.878215178124995832, -5.746835883940462963, 0.2906249993854838065 ) ) ;
#9085=CYLINDRICAL_SURFACE ( 'NONE', #18846, 4.000000000000000000 ) ;
#9122=CARTESIAN_POINT ( 'NONE',  ( 3.735045420075836212E-15, -4.662447845253954171, 0.2531249993854848279 ) ) ;
#9128=ADVANCED_FACE ( 'NONE', ( #12131 ), #6627, .T. ) ;
#9136=EDGE_CURVE ( 'NONE', #17175, #15910, #8090, .T. ) ;
#9158=DIRECTION ( 'NONE',  ( -1.000000000000000000, 0.000000000000000000, 0.000000000000000000 ) ) ;
#9161=CARTESIAN_POINT ( 'NONE',  ( -3.756430356249995661, -6.831223922626973533, 4.490624999385484095 ) ) ;
#9162=CARTESIAN_POINT ( 'NONE',  ( -3.999999999999996447, -8.999999999999992895, 1.968749998770967569 ) ) ;
#9169=CARTESIAN_POINT ( 'NONE',  ( 3.756430356250003655, -8.999999999999992895, 4.640624999385483562 ) ) ;
#9175=CARTESIAN_POINT ( 'NONE',  ( 3.756430356250003655, -8.999999999999992895, 4.753124999385485161 ) ) ;
#9234=CARTESIAN_POINT ( 'NONE',  ( -3.999999999999996447, -8.999999999999992895, 2.024999999999999023 ) ) ;
#9267=CARTESIAN_POINT ( 'NONE',  ( 1.878215178125000939, -12.25316411605952283, 1.865624999385483873 ) ) ;
#9275=CARTESIAN_POINT ( 'NONE',  ( -3.999999999999996447, -8.999999999999992895, 18.00000000000000000 ) ) ;
#9303=CARTESIAN_POINT ( 'NONE',  ( 3.735045420075836212E-15, -4.662447845253954171, 1.603124999385479921 ) ) ;
#9304=CARTESIAN_POINT ( 'NONE',  ( -3.999999999999997335, -11.30940107675849404, 1.556249998770965037 ) ) ;
#9308=CARTESIAN_POINT ( 'NONE',  ( 3.735045420075836212E-15, -4.662447845253954171, 3.403124999385483296 ) ) ;
#9313=CARTESIAN_POINT ( 'NONE',  ( -1.878215178124998497, -12.25316411605951927, 4.153124999385485516 ) ) ;
#9320=DIRECTION ( 'NONE',  ( 0.000000000000000000, 0.000000000000000000, 1.000000000000000000 ) ) ;
#9322=AXIS2_PLACEMENT_3D ( 'NONE', #16074, #1691, #11611 ) ;
#9327=VERTEX_POINT ( 'NONE', #25324 ) ;
#9331=VERTEX_POINT ( 'NONE', #11577 ) ;
#9421=CARTESIAN_POINT ( 'NONE',  ( -3.999999999999996447, -8.999999999999992895, 1.068749998770966103 ) ) ;
#9424=CARTESIAN_POINT ( 'NONE',  ( -1.878215178124995832, -5.746835883940462963, 2.990624999385481431 ) ) ;
#9425=CARTESIAN_POINT ( 'NONE',  ( -3.999999999999996447, -8.999999999999992895, 2.868749998770965703 ) ) ;
#9428=CARTESIAN_POINT ( 'NONE',  ( 2.620986760973688460E-15, -13.61880215351699874, 3.881249998770965437 ) ) ;
#9430=CARTESIAN_POINT ( 'NONE',  ( -1.999999999999995781, -5.535898384862237620, 1.500000000000001332 ) ) ;
#9436=CARTESIAN_POINT ( 'NONE',  ( 1.878215178125000939, -12.25316411605952283, 4.228124999385483918 ) ) ;
#9438=CARTESIAN_POINT ( 'NONE',  ( -3.999999999999996447, -8.999999999999992895, 3.318749998770968102 ) ) ;
#9468=ORIENTED_EDGE ( 'NONE', *, *, #9005, .T. ) ;
#9471=ADVANCED_FACE ( 'NONE', ( #7367 ), #18890, .T. ) ;
#9474=CARTESIAN_POINT ( 'NONE',  ( -3.999999999999996447, -8.999999999999992895, 4.275000000000001243 ) ) ;
#9508=CARTESIAN_POINT ( 'NONE',  ( 3.735045420075836212E-15, -4.662447845253954171, 0.7031249993854805647 ) ) ;
#9510=CARTESIAN_POINT ( 'NONE',  ( 3.756430356250004099, -6.831223922626973533, 3.440624999385483829 ) ) ;
#9537=ORIENTED_EDGE ( 'NONE', *, *, #18300, .F. ) ;
#9543=CARTESIAN_POINT ( 'NONE',  ( 3.756430356250004099, -6.831223922626973533, 2.428124999385481431 ) ) ;
#9544=CARTESIAN_POINT ( 'NONE',  ( 4.000000000000003553, -6.690598923241489970, 2.231249998770966858 ) ) ;
#9546=CARTESIAN_POINT ( 'NONE',  ( 3.999999999999987121, -11.30940107675850648, 3.956249998770966947 ) ) ;
#9549=CARTESIAN_POINT ( 'NONE',  ( -1.999999999999995781, -5.535898384862237620, 1.950000000000000400 ) ) ;
#9551=FACE_OUTER_BOUND ( 'NONE', #162, .T. ) ;
#9557=CARTESIAN_POINT ( 'NONE',  ( 2.000000000000000888, -12.46410161513774817, 4.818749998770965881 ) ) ;
#9626=AXIS2_PLACEMENT_3D ( 'NONE', #1485, #19393, #21104 ) ;
#9643=CARTESIAN_POINT ( 'NONE',  ( 3.756430356250003655, -8.999999999999992895, 0.5906249993854819635 ) ) ;
#9655=LINE ( 'NONE', #9275, #17451 ) ;
#9663=CARTESIAN_POINT ( 'NONE',  ( 3.752267015613588906E-15, -4.381197846482986158, 2.362499999999997602 ) ) ;
#9683=CARTESIAN_POINT ( 'NONE',  ( -1.878215178124998497, -12.25316411605951927, 3.140624999385482230 ) ) ;
#9684=CARTESIAN_POINT ( 'NONE',  ( 2.000000000000000888, -12.46410161513774817, 2.118749998770968368 ) ) ;
#9688=ADVANCED_FACE ( 'NONE', ( #6048 ), #13524, .T. ) ;
#9691=CARTESIAN_POINT ( 'NONE',  ( -3.999999999999996003, -6.690598923241487306, 1.537500000000000089 ) ) ;
#9717=CARTESIAN_POINT ( 'NONE',  ( 3.756430356250003655, -8.999999999999992895, 0.2531249993854844949 ) ) ;
#9748=CARTESIAN_POINT ( 'NONE',  ( -3.999999999999996447, -8.999999999999992895, 1.068749998770966103 ) ) ;
#9755=( BOUNDED_CURVE ( )  B_SPLINE_CURVE ( 2, ( #22099, #4188, #5757, #20264, #18194, #279, #14011 ),
 .UNSPECIFIED., .F., .F. ) 
 B_SPLINE_CURVE_WITH_KNOTS ( ( 3, 2, 2, 3 ),
 ( 0.3500000000000000888, 0.3666666666666666963, 0.3833333333333333592, 0.3999999999999999667 ),
 .UNSPECIFIED. ) 
 CURVE ( )  GEOMETRIC_REPRESENTATION_ITEM ( )  RATIONAL_B_SPLINE_CURVE ( ( 0.9999999999999991118, 0.8660254037844395958, 1.000000000000000000, 0.8660254037844387076, 1.000000000000000000, 0.8660254037844391517, 0.9999999999999995559 ) ) 
 REPRESENTATION_ITEM ( '' )  );
#9765=EDGE_CURVE ( 'NONE', #5385, #13208, #6555, .T. ) ;
#9775=CARTESIAN_POINT ( 'NONE',  ( 3.756430356250003211, -6.831223922626973533, 3.328124999385480898 ) ) ;
#9789=ADVANCED_FACE ( 'NONE', ( #12716 ), #14537, .T. ) ;
#9799=ORIENTED_EDGE ( 'NONE', *, *, #7902, .F. ) ;
#9807=CARTESIAN_POINT ( 'NONE',  ( 3.735045420075836212E-15, -4.662447845253954171, 2.503124999385483385 ) ) ;
#9808=CARTESIAN_POINT ( 'NONE',  ( 2.000000000000003997, -5.535898384862238508, 3.168749998770967302 ) ) ;
#9813=CARTESIAN_POINT ( 'NONE',  ( -1.999999999999995781, -5.535898384862237620, 1.049999999999998934 ) ) ;
#9824=ORIENTED_EDGE ( 'NONE', *, *, #24086, .T. ) ;
#9827=ORIENTED_EDGE ( 'NONE', *, *, #12249, .F. ) ;
#9836=CARTESIAN_POINT ( 'NONE',  ( -1.878215178124995832, -5.746835883940462963, 0.4031249993854852942 ) ) ;
#9858=ORIENTED_EDGE ( 'NONE', *, *, #15600, .T. ) ;
#9892=CARTESIAN_POINT ( 'NONE',  ( 3.735045420075836212E-15, -4.662447845253954171, 4.303124999385482319 ) ) ;
#9899=FACE_OUTER_BOUND ( 'NONE', #16336, .T. ) ;
#9907=LINE ( 'NONE', #23393, #12042 ) ;
#9917=ORIENTED_EDGE ( 'NONE', *, *, #4034, .F. ) ;
#9924=CARTESIAN_POINT ( 'NONE',  ( 3.756430356250002323, -11.16877607737301226, 2.353124999385479477 ) ) ;
#9925=CARTESIAN_POINT ( 'NONE',  ( 4.000000000000003553, -6.690598923241489970, 4.481249998770969079 ) ) ;
#9931=CARTESIAN_POINT ( 'NONE',  ( -3.999999999999996003, -6.690598923241487306, 1.987499999999999600 ) ) ;
#9948=CARTESIAN_POINT ( 'NONE',  ( -3.999999999999996447, -8.999999999999992895, 1.518749998770968501 ) ) ;
#9958=CARTESIAN_POINT ( 'NONE',  ( -3.756430356249997882, -11.16877607737301226, 1.415624999385483029 ) ) ;
#10019=CARTESIAN_POINT ( 'NONE',  ( -3.756430356249997438, -11.16877607737301048, 4.453124999385482674 ) ) ;
#10039=DIRECTION ( 'NONE',  ( -0.000000000000000000, -0.000000000000000000, -1.000000000000000000 ) ) ;
#10048=VERTEX_POINT ( 'NONE', #18686 ) ;
#10058=CARTESIAN_POINT ( 'NONE',  ( 4.000000000000001776, -11.30940107675849760, 4.856249998770966414 ) ) ;
#10080=CARTESIAN_POINT ( 'NONE',  ( 3.469446951953614189E-15, -8.999999999999992895, 18.00000000000000000 ) ) ;
#10090=CARTESIAN_POINT ( 'NONE',  ( -3.756430356249996994, -8.999999999999992895, 0.4781249993854840286 ) ) ;
#10097=CARTESIAN_POINT ( 'NONE',  ( 1.878215178125004048, -5.746835883940462963, 1.115624999385483207 ) ) ;
#10111=DIRECTION ( 'NONE',  ( 0.000000000000000000, 0.000000000000000000, 1.000000000000000000 ) ) ;
#10116=EDGE_CURVE ( 'NONE', #4330, #7795, #13445, .T. ) ;
#10120=ORIENTED_EDGE ( 'NONE', *, *, #19273, .T. ) ;
#10135=CARTESIAN_POINT ( 'NONE',  ( 4.000000000000003553, -8.999999999999992895, 18.00000000000000000 ) ) ;
#10152=CARTESIAN_POINT ( 'NONE',  ( -3.756430356249996105, -6.831223922626973533, 3.028124999385485072 ) ) ;
#10185=CARTESIAN_POINT ( 'NONE',  ( 3.752267015613588906E-15, -4.381197846482986158, 3.206249998770963838 ) ) ;
#10190=CARTESIAN_POINT ( 'NONE',  ( 2.000000000000000888, -12.46410161513774817, 1.668749998770965970 ) ) ;
#10193=PLANE ( 'NONE',  #14547 ) ;
#10214=CARTESIAN_POINT ( 'NONE',  ( -3.756430356249995661, -6.831223922626973533, 2.240624999385484539 ) ) ;
#10218=CARTESIAN_POINT ( 'NONE',  ( 3.469446951953614189E-15, -8.999999999999992895, 18.00000000000000000 ) ) ;
#10220=CARTESIAN_POINT ( 'NONE',  ( 3.756430356250002323, -11.16877607737301226, 0.5531249993854806535 ) ) ;
#10225=DIRECTION ( 'NONE',  ( -1.000000000000000000, 0.000000000000000000, 0.000000000000000000 ) ) ;
#10226=VERTEX_POINT ( 'NONE', #23138 ) ;
#10234=CIRCLE ( 'NONE', #21932, 3.000000000000000444 ) ;
#10236=ORIENTED_EDGE ( 'NONE', *, *, #12394, .T. ) ;
#10252=CARTESIAN_POINT ( 'NONE',  ( 3.752267015613588906E-15, -4.381197846482986158, 4.556249998770967480 ) ) ;
#10255=CARTESIAN_POINT ( 'NONE',  ( -3.999999999999996447, -8.999999999999992895, 0.2249999999999995060 ) ) ;
#10270=CARTESIAN_POINT ( 'NONE',  ( -3.756430356249996105, -6.831223922626973533, 3.928124999385480542 ) ) ;
#10275=( BOUNDED_CURVE ( )  B_SPLINE_CURVE ( 2, ( #19306, #11842, #11457, #23735, #25443, #3869, #1403 ),
 .UNSPECIFIED., .F., .F. ) 
 B_SPLINE_CURVE_WITH_KNOTS ( ( 3, 2, 2, 3 ),
 ( 0.5499999999999997113, 0.5666666666666665408, 0.5833333333333335924, 0.6000000000000004219 ),
 .UNSPECIFIED. ) 
 CURVE ( )  GEOMETRIC_REPRESENTATION_ITEM ( )  RATIONAL_B_SPLINE_CURVE ( ( 1.000000000000002665, 0.8660254037844360431, 1.000000000000000000, 0.8660254037844387076, 1.000000000000000000, 0.8660254037844351549, 1.000000000000003553 ) ) 
 REPRESENTATION_ITEM ( '' )  );
#10304=CARTESIAN_POINT ( 'NONE',  ( 3.756430356250004099, -6.831223922626973533, 0.7406249993854815417 ) ) ;
#10322=CARTESIAN_POINT ( 'NONE',  ( -3.999999999999996447, -8.999999999999992895, 3.768749998770966947 ) ) ;
#10333=CARTESIAN_POINT ( 'NONE',  ( 3.756430356250003655, -8.999999999999992895, 3.403124999385484628 ) ) ;
#10337=CARTESIAN_POINT ( 'NONE',  ( 3.735045420075836212E-15, -4.662447845253954171, 0.7031249993854805647 ) ) ;
#10341=CARTESIAN_POINT ( 'NONE',  ( -1.878215178124995832, -5.746835883940462963, 1.753124999385485827 ) ) ;
#10374=ADVANCED_FACE ( 'NONE', ( #8205 ), #3759, .T. ) ;
#10424=ORIENTED_EDGE ( 'NONE', *, *, #7955, .T. ) ;
#10437=VECTOR ( 'NONE', #11778, 1000.000000000000000 ) ;
#10440=CARTESIAN_POINT ( 'NONE',  ( 3.756430356250002323, -11.16877607737301226, 2.915624999385482141 ) ) ;
#10462=ORIENTED_EDGE ( 'NONE', *, *, #16679, .T. ) ;
#10472=CARTESIAN_POINT ( 'NONE',  ( 1.878215178125000939, -12.25316411605952283, 1.978124999385485250 ) ) ;
#10480=CARTESIAN_POINT ( 'NONE',  ( 1.878215178125000939, -12.25316411605952283, 1.865624999385483873 ) ) ;
#10485=CARTESIAN_POINT ( 'NONE',  ( 3.735045420075836212E-15, -4.662447845253954171, 1.265624999385483118 ) ) ;
#10515=CARTESIAN_POINT ( 'NONE',  ( 2.620986760973688460E-15, -13.61880215351699874, 2.137499999999999734 ) ) ;
#10521=CARTESIAN_POINT ( 'NONE',  ( -4.000000000000010658, -6.690598923241495299, 1.537500000000000311 ) ) ;
#10522=ORIENTED_EDGE ( 'NONE', *, *, #19096, .F. ) ;
#10539=CARTESIAN_POINT ( 'NONE',  ( 3.999999999999972466, -6.690598923241471319, 3.187499999999999556 ) ) ;
#10569=CARTESIAN_POINT ( 'NONE',  ( 2.000000000000000888, -12.46410161513774817, 3.468749998770968901 ) ) ;
#10571=CARTESIAN_POINT ( 'NONE',  ( 3.735045420075836212E-15, -4.662447845253954171, 1.265624999385483118 ) ) ;
#10589=EDGE_CURVE ( 'NONE', #13396, #6968, #22524, .T. ) ;
#10591=CARTESIAN_POINT ( 'NONE',  ( -1.999999999999995781, -5.535898384862237620, 3.693749998770968546 ) ) ;
#10605=CARTESIAN_POINT ( 'NONE',  ( -3.756430356249995661, -6.831223922626973533, 3.140624999385484006 ) ) ;
#10611=CARTESIAN_POINT ( 'NONE',  ( 3.756430356250004099, -6.831223922626973533, 1.978124999385481697 ) ) ;
#10615=CARTESIAN_POINT ( 'NONE',  ( 1.878215178125000939, -12.25316411605952283, 1.078124999385483784 ) ) ;
#10623=FACE_BOUND ( 'NONE', #19524, .T. ) ;
#10638=EDGE_CURVE ( 'NONE', #6033, #13093, #4996, .T. ) ;
#10644=CARTESIAN_POINT ( 'NONE',  ( -4.000000000000010658, -11.30940107675848694, 0.2624999999999985678 ) ) ;
#10648=CARTESIAN_POINT ( 'NONE',  ( -3.756430356249997882, -11.16877607737301226, 0.4031249993854806868 ) ) ;
#10650=ORIENTED_EDGE ( 'NONE', *, *, #5566, .T. ) ;
#10651=CARTESIAN_POINT ( 'NONE',  ( 4.000000000000003553, -8.999999999999992895, 4.443749998770965881 ) ) ;
#10671=DIRECTION ( 'NONE',  ( -1.000000000000000000, 0.000000000000000000, 0.000000000000000000 ) ) ;
#10674=VERTEX_POINT ( 'NONE', #16913 ) ;
#10676=CARTESIAN_POINT ( 'NONE',  ( -3.999999999999996447, -8.999999999999992895, 1.125000000000000888 ) ) ;
#10688=ORIENTED_EDGE ( 'NONE', *, *, #24086, .F. ) ;
#10695=CARTESIAN_POINT ( 'NONE',  ( 3.756430356250004099, -6.831223922626973533, 2.090624999385480631 ) ) ;
#10724=CARTESIAN_POINT ( 'NONE',  ( -1.878215178124995832, -5.746835883940462963, 3.553124999385485427 ) ) ;
#10730=CARTESIAN_POINT ( 'NONE',  ( 1.878215178125000939, -12.25316411605952283, 3.215624999385484184 ) ) ;
#10736=CARTESIAN_POINT ( 'NONE',  ( -3.756430356249996994, -8.999999999999992895, 0.9281249993854829849 ) ) ;
#10746=ORIENTED_EDGE ( 'NONE', *, *, #18146, .F. ) ;
#10765=CARTESIAN_POINT ( 'NONE',  ( -4.000000000000026645, -6.690598923241505958, 3.281249998770966680 ) ) ;
#10769=CARTESIAN_POINT ( 'NONE',  ( 4.000000000000003553, -8.999999999999992895, 0.4499999999999990119 ) ) ;
#10785=CARTESIAN_POINT ( 'NONE',  ( -1.878215178124998497, -12.25316411605951927, 4.490624999385482319 ) ) ;
#10820=CARTESIAN_POINT ( 'NONE',  ( -3.999999999999996447, -8.999999999999992895, 2.024999999999999023 ) ) ;
#10824=CARTESIAN_POINT ( 'NONE',  ( -1.878215178124998497, -12.25316411605951927, 2.803124999385484539 ) ) ;
#10841=CARTESIAN_POINT ( 'NONE',  ( 3.469446951953614189E-15, -8.999999999999992895, 18.00000000000000000 ) ) ;
#10858=CARTESIAN_POINT ( 'NONE',  ( 3.735045420075836212E-15, -4.662447845253954171, 4.415624999385481253 ) ) ;
#10862=CARTESIAN_POINT ( 'NONE',  ( -1.999999999999998224, -12.46410161513774639, 0.3000000000000016542 ) ) ;
#10868=CARTESIAN_POINT ( 'NONE',  ( 1.878215178125004048, -5.746835883940462963, 2.578124999385485339 ) ) ;
#10877=ORIENTED_EDGE ( 'NONE', *, *, #13602, .T. ) ;
#10901=DIRECTION ( 'NONE',  ( 0.000000000000000000, 0.000000000000000000, 1.000000000000000000 ) ) ;
#10964=CARTESIAN_POINT ( 'NONE',  ( -3.756430356249995661, -6.831223922626973533, 1.340624999385481075 ) ) ;
#11000=CARTESIAN_POINT ( 'NONE',  ( 3.735045420075836212E-15, -4.662447845253954171, 1.153124999385480187 ) ) ;
#11005=CARTESIAN_POINT ( 'NONE',  ( -1.999999999999995781, -5.535898384862237620, 0.5999999999999998668 ) ) ;
#11006=CARTESIAN_POINT ( 'NONE',  ( -3.756430356249995661, -6.831223922626973533, 3.478124999385480809 ) ) ;
#11008=DIRECTION ( 'NONE',  ( -0.000000000000000000, -0.000000000000000000, -1.000000000000000000 ) ) ;
#11011=CARTESIAN_POINT ( 'NONE',  ( -3.756430356249996105, -6.831223922626973533, 3.590624999385483740 ) ) ;
#11055=ADVANCED_FACE ( 'NONE', ( #6622 ), #20626, .T. ) ;
#11072=LINE ( 'NONE', #14491, #12183 ) ;
#11085=CARTESIAN_POINT ( 'NONE',  ( 2.672651547586948120E-15, -13.33755215474603162, 0.9281249993854823188 ) ) ;
#11086=EDGE_CURVE ( 'NONE', #23657, #9327, #14612, .T. ) ;
#11118=CARTESIAN_POINT ( 'NONE',  ( -1.878215178124998497, -12.25316411605951927, 1.340624999385482630 ) ) ;
#11119=CARTESIAN_POINT ( 'NONE',  ( -3.999999999999996003, -6.690598923241487306, 1.481249998770963083 ) ) ;
#11125=CARTESIAN_POINT ( 'NONE',  ( 4.000000000000003553, -6.690598923241489970, 0.4874999999999966582 ) ) ;
#11127=LINE ( 'NONE', #19486, #7858 ) ;
#11195=ORIENTED_EDGE ( 'NONE', *, *, #20514, .F. ) ;
#11197=ORIENTED_EDGE ( 'NONE', *, *, #16724, .T. ) ;
#11201=ORIENTED_EDGE ( 'NONE', *, *, #11664, .F. ) ;
#11206=CARTESIAN_POINT ( 'NONE',  ( -1.878215178124998497, -12.25316411605951927, 1.790624999385481697 ) ) ;
#11209=CARTESIAN_POINT ( 'NONE',  ( 3.735045420075836212E-15, -4.662447845253954171, 3.515624999385486227 ) ) ;
#11224=CARTESIAN_POINT ( 'NONE',  ( 2.620986760973688460E-15, -13.61880215351699874, 4.387499999999998401 ) ) ;
#11226=ORIENTED_EDGE ( 'NONE', *, *, #21962, .T. ) ;
#11243=CARTESIAN_POINT ( 'NONE',  ( 3.756430356250004099, -6.831223922626973533, 1.528124999385482186 ) ) ;
#11244=CARTESIAN_POINT ( 'NONE',  ( 3.752267015613588906E-15, -4.381197846482986158, 0.9562499987709653926 ) ) ;
#11249=CARTESIAN_POINT ( 'NONE',  ( -3.756430356249996994, -8.999999999999992895, 3.515624999385482674 ) ) ;
#11254=CARTESIAN_POINT ( 'NONE',  ( -3.999999999999996447, -8.999999999999992895, 0.6187499987709670357 ) ) ;
#11284=CLOSED_SHELL ( 'NONE', ( #12038, #9688, #768, #3593, #13380, #10374, #14284, #18654, #13137, #15455, #277, #9471, #20955, #9789, #14218, #18958, #11055, #21598, #12615, #6535, #9128, #13964, #15442, #22657, #20318, #1422, #18176, #3689, #17943, #6556, #22136 ) ) ;
#11289=ORIENTED_EDGE ( 'NONE', *, *, #16237, .F. ) ;
#11292=VERTEX_POINT ( 'NONE', #5440 ) ;
#11345=CARTESIAN_POINT ( 'NONE',  ( 1.878215178125004048, -5.746835883940462963, 2.015624999385484450 ) ) ;
#11363=LINE ( 'NONE', #15560, #1218 ) ;
#11383=CARTESIAN_POINT ( 'NONE',  ( 3.756430356250003655, -8.999999999999992895, 2.390624999385481342 ) ) ;
#11384=CARTESIAN_POINT ( 'NONE',  ( -3.999999999999997335, -11.30940107675849404, 2.456249998770964726 ) ) ;
#11390=CARTESIAN_POINT ( 'NONE',  ( -3.999999999999996003, -6.690598923241487306, 1.087499999999996358 ) ) ;
#11391=CARTESIAN_POINT ( 'NONE',  ( 4.000000000000003553, -8.999999999999992895, 18.00000000000000000 ) ) ;
#11396=CARTESIAN_POINT ( 'NONE',  ( 3.735045420075836212E-15, -4.662447845253954171, 3.965624999385486404 ) ) ;
#11397=DIRECTION ( 'NONE',  ( 1.000000000000000000, 0.000000000000000000, 0.000000000000000000 ) ) ;
#11442=( BOUNDED_CURVE ( )  B_SPLINE_CURVE ( 2, ( #404, #2360, #16221, #18311, #22488, #20531, #6147 ),
 .UNSPECIFIED., .F., .F. ) 
 B_SPLINE_CURVE_WITH_KNOTS ( ( 3, 2, 2, 3 ),
 ( 0.6000000000000004219, 0.6166666666666670293, 0.6333333333333336368, 0.6500000000000002442 ),
 .UNSPECIFIED. ) 
 CURVE ( )  GEOMETRIC_REPRESENTATION_ITEM ( )  RATIONAL_B_SPLINE_CURVE ( ( 0.9999999999999964473, 0.8660254037844422603, 1.000000000000000000, 0.8660254037844387076, 1.000000000000000000, 0.8660254037844369313, 1.000000000000001776 ) ) 
 REPRESENTATION_ITEM ( '' )  );
#11447=EDGE_CURVE ( 'NONE', #21005, #523, #74, .T. ) ;
#11457=CARTESIAN_POINT ( 'NONE',  ( -1.999999999999998224, -12.46410161513774639, 2.943749998770967657 ) ) ;
#11475=CARTESIAN_POINT ( 'NONE',  ( -3.756430356249996994, -8.999999999999992895, 0.3656249993854825409 ) ) ;
#11476=CARTESIAN_POINT ( 'NONE',  ( 2.672651547586948120E-15, -13.33755215474602984, 4.640624999385483562 ) ) ;
#11507=CARTESIAN_POINT ( 'NONE',  ( 3.735045420075836212E-15, -4.662447845253954171, 2.953124999385479565 ) ) ;
#11508=CARTESIAN_POINT ( 'NONE',  ( -1.999999999999995781, -5.535898384862237620, 2.793749998770966858 ) ) ;
#11514=CARTESIAN_POINT ( 'NONE',  ( -3.999999999999996447, -8.999999999999992895, 0.6749999999999984901 ) ) ;
#11522=CARTESIAN_POINT ( 'NONE',  ( -3.999999999999996447, -8.999999999999992895, 4.668749998770968190 ) ) ;
#11535=EDGE_CURVE ( 'NONE', #9331, #12074, #2800, .T. ) ;
#11538=CARTESIAN_POINT ( 'NONE',  ( -3.756430356249997882, -11.16877607737301226, 0.9656249993854834068 ) ) ;
#11561=CARTESIAN_POINT ( 'NONE',  ( -3.999999999999996447, -8.999999999999992895, 4.218749998770966236 ) ) ;
#11574=( BOUNDED_CURVE ( )  B_SPLINE_CURVE ( 2, ( #6881, #10539, #24802, #6611, #14357, #4276, #12251 ),
 .UNSPECIFIED., .F., .T. ) 
 B_SPLINE_CURVE_WITH_KNOTS ( ( 3, 2, 2, 3 ),
 ( 0.7000000000000001776, 0.7166666666666667851, 0.7333333333333333925, 0.7500000000000000000 ),
 .UNSPECIFIED. ) 
 CURVE ( )  GEOMETRIC_REPRESENTATION_ITEM ( )  RATIONAL_B_SPLINE_CURVE ( ( 0.9999999999999982236, 0.8660254037844404840, 1.000000000000000000, 0.8660254037844387076, 1.000000000000000000, 0.8660254037844387076, 1.000000000000000000 ) ) 
 REPRESENTATION_ITEM ( '' )  );
#11577=CARTESIAN_POINT ( 'NONE',  ( 4.000000000000003553, -8.999999999999992895, 0.000000000000000000 ) ) ;
#11593=CARTESIAN_POINT ( 'NONE',  ( 3.756430356250002323, -11.16877607737301403, 1.003124999385480498 ) ) ;
#11597=DIRECTION ( 'NONE',  ( -0.000000000000000000, -0.000000000000000000, -1.000000000000000000 ) ) ;
#11610=CARTESIAN_POINT ( 'NONE',  ( -1.999999999999998224, -12.46410161513774639, 4.349999999999999645 ) ) ;
#11611=DIRECTION ( 'NONE',  ( 1.000000000000000000, 0.000000000000000000, 0.000000000000000000 ) ) ;
#11630=CARTESIAN_POINT ( 'NONE',  ( 3.756430356250002323, -11.16877607737301226, 3.253124999385482941 ) ) ;
#11631=CARTESIAN_POINT ( 'NONE',  ( 4.000000000000003553, -6.690598923241489970, 1.781249998770966680 ) ) ;
#11637=CARTESIAN_POINT ( 'NONE',  ( 3.752267015613588906E-15, -4.381197846482986158, 2.812499999999997335 ) ) ;
#11645=AXIS2_PLACEMENT_3D ( 'NONE', #10841, #543, #6805 ) ;
#11646=CARTESIAN_POINT ( 'NONE',  ( -3.999999999999936051, -11.30940107675852779, 4.706249998770969611 ) ) ;
#11663=VECTOR ( 'NONE', #19814, 1000.000000000000000 ) ;
#11664=EDGE_CURVE ( 'NONE', #5385, #24155, #3573, .T. ) ;
#11665=CARTESIAN_POINT ( 'NONE',  ( 1.878215178125004048, -5.746835883940462963, 0.7781249993854856273 ) ) ;
#11673=AXIS2_PLACEMENT_3D ( 'NONE', #13282, #25056, #5432 ) ;
#11702=CARTESIAN_POINT ( 'NONE',  ( 4.000000000000003553, -8.999999999999992895, 0.000000000000000000 ) ) ;
#11709=CARTESIAN_POINT ( 'NONE',  ( -3.999999999999996447, -8.999999999999992895, 4.668749998770968190 ) ) ;
#11730=CARTESIAN_POINT ( 'NONE',  ( -1.878215178124995832, -5.746835883940462963, 3.440624999385483829 ) ) ;
#11768=CARTESIAN_POINT ( 'NONE',  ( -1.878215178124998497, -12.25316411605951927, 2.690624999385483385 ) ) ;
#11769=CARTESIAN_POINT ( 'NONE',  ( 4.000000000000003553, -8.999999999999992895, 3.993749998770966592 ) ) ;
#11776=CARTESIAN_POINT ( 'NONE',  ( -1.999999999999998224, -12.46410161513774639, 2.550000000000000266 ) ) ;
#11778=DIRECTION ( 'NONE',  ( -0.000000000000000000, -0.000000000000000000, -1.000000000000000000 ) ) ;
#11796=ORIENTED_EDGE ( 'NONE', *, *, #11977, .F. ) ;
#11797=CARTESIAN_POINT ( 'NONE',  ( -3.999999999999996447, -8.999999999999992895, 2.868749998770965703 ) ) ;
#11806=DIRECTION ( 'NONE',  ( -0.000000000000000000, -0.000000000000000000, -1.000000000000000000 ) ) ;
#11811=CARTESIAN_POINT ( 'NONE',  ( 1.878215178125000939, -12.25316411605952283, 0.6281249993854848279 ) ) ;
#11827=CARTESIAN_POINT ( 'NONE',  ( -1.999999999999995781, -5.535898384862237620, 4.199999999999999289 ) ) ;
#11842=CARTESIAN_POINT ( 'NONE',  ( -4.000000000000043521, -11.30940107675846562, 2.906249998770967125 ) ) ;
#11860=CARTESIAN_POINT ( 'NONE',  ( 3.735045420075836212E-15, -4.662447845253954171, 2.953124999385479121 ) ) ;
#11893=CARTESIAN_POINT ( 'NONE',  ( 3.756430356250002323, -11.16877607737301226, 2.803124999385479210 ) ) ;
#11894=CARTESIAN_POINT ( 'NONE',  ( 4.000000000000001776, -11.30940107675849760, 3.956249998770966947 ) ) ;
#11899=CARTESIAN_POINT ( 'NONE',  ( -3.999999999999996447, -8.999999999999992895, 2.925000000000000711 ) ) ;
#11908=EDGE_LOOP ( 'NONE', ( #21246, #12200, #9858 ) ) ;
#11910=CARTESIAN_POINT ( 'NONE',  ( 4.000000000000003553, -8.999999999999992895, 18.00000000000000000 ) ) ;
#11922=DIRECTION ( 'NONE',  ( -1.000000000000000000, 0.000000000000000000, 0.000000000000000000 ) ) ;
#11929=CARTESIAN_POINT ( 'NONE',  ( 3.756430356250003211, -6.831223922626973533, 0.7406249993854815417 ) ) ;
#11948=CARTESIAN_POINT ( 'NONE',  ( 3.756430356250003655, -8.999999999999992895, 0.2531249993854844949 ) ) ;
#11971=CARTESIAN_POINT ( 'NONE',  ( 3.469446951953614189E-15, -8.999999999999992895, 18.00000000000000000 ) ) ;
#11976=CARTESIAN_POINT ( 'NONE',  ( -3.756430356249996105, -6.831223922626973533, 2.578124999385481342 ) ) ;
#11977=EDGE_CURVE ( 'NONE', #14884, #1313, #11072, .T. ) ;
#11979=FILL_AREA_STYLE ('',( #22052 ) ) ;
#11980=CARTESIAN_POINT ( 'NONE',  ( -3.999999999999996447, -8.999999999999992895, 0.6749999999999984901 ) ) ;
#11999=ORIENTED_EDGE ( 'NONE', *, *, #18697, .F. ) ;
#12010=CARTESIAN_POINT ( 'NONE',  ( -1.999999999999998224, -12.46410161513774639, 3.843749998770965792 ) ) ;
#12036=ORIENTED_EDGE ( 'NONE', *, *, #10116, .F. ) ;
#12038=ADVANCED_FACE ( 'NONE', ( #23358 ), #3610, .F. ) ;
#12042=VECTOR ( 'NONE', #17768, 999.9999999999998863 ) ;
#12050=CARTESIAN_POINT ( 'NONE',  ( 3.756430356250003655, -8.999999999999992895, 1.940624999385482496 ) ) ;
#12053=CARTESIAN_POINT ( 'NONE',  ( 4.000000000000003553, -8.999999999999992895, 3.599999999999999201 ) ) ;
#12074=VERTEX_POINT ( 'NONE', #2148 ) ;
#12113=CARTESIAN_POINT ( 'NONE',  ( 3.756430356250002323, -11.16877607737301403, 2.803124999385479654 ) ) ;
#12118=( BOUNDED_CURVE ( )  B_SPLINE_CURVE ( 2, ( #8365, #16092, #19866, #17916, #7983, #6403, #15971 ),
 .UNSPECIFIED., .F., .F. ) 
 B_SPLINE_CURVE_WITH_KNOTS ( ( 3, 2, 2, 3 ),
 ( 0.1499999999999996891, 0.1666666666666665741, 0.1833333333333334592, 0.2000000000000003719 ),
 .UNSPECIFIED. ) 
 CURVE ( )  GEOMETRIC_REPRESENTATION_ITEM ( )  RATIONAL_B_SPLINE_CURVE ( ( 1.000000000000002665, 0.8660254037844363761, 1.000000000000000000, 0.8660254037844387076, 1.000000000000000000, 0.8660254037844358210, 1.000000000000002887 ) ) 
 REPRESENTATION_ITEM ( '' )  );
#12120=CARTESIAN_POINT ( 'NONE',  ( 4.000000000000003553, -8.999999999999992895, 18.00000000000000000 ) ) ;
#12123=CYLINDRICAL_SURFACE ( 'NONE', #14560, 4.000000000000000000 ) ;
#12131=FACE_OUTER_BOUND ( 'NONE', #25303, .T. ) ;
#12136=LINE ( 'NONE', #14494, #25027 ) ;
#12142=PRODUCT ( 'stem', 'stem', '', ( #13163 ) ) ;
#12152=CARTESIAN_POINT ( 'NONE',  ( -3.999999999999996447, -8.999999999999992895, 3.318749998770968102 ) ) ;
#12158=CARTESIAN_POINT ( 'NONE',  ( 4.000000000000003553, -8.999999999999992895, 4.049999999999998046 ) ) ;
#12168=CARTESIAN_POINT ( 'NONE',  ( 3.999999999999972466, -6.690598923241471319, 3.581249998770966503 ) ) ;
#12183=VECTOR ( 'NONE', #6507, 1000.000000000000000 ) ;
#12185=CARTESIAN_POINT ( 'NONE',  ( -3.756430356249997882, -11.16877607737301226, 1.865624999385482985 ) ) ;
#12193=CARTESIAN_POINT ( 'NONE',  ( -3.756430356249997882, -11.16877607737301226, 2.203124999385479565 ) ) ;
#12195=CARTESIAN_POINT ( 'NONE',  ( 3.878215178125003604, -8.999999999999992895, 4.570312499692741781 ) ) ;
#12200=ORIENTED_EDGE ( 'NONE', *, *, #13246, .F. ) ;
#12226=CARTESIAN_POINT ( 'NONE',  ( -4.000000000000021316, -11.30940107675847806, 2.062499999999996891 ) ) ;
#12231=CARTESIAN_POINT ( 'NONE',  ( -1.999999999999998224, -12.46410161513774639, 0.3000000000000016542 ) ) ;
#12240=PLANE ( 'NONE',  #17563 ) ;
#12247=CARTESIAN_POINT ( 'NONE',  ( 3.756430356250003655, -8.999999999999992895, 3.740624999385481875 ) ) ;
#12249=EDGE_CURVE ( 'NONE', #13593, #702, #17411, .T. ) ;
#12251=CARTESIAN_POINT ( 'NONE',  ( -3.999999999999996447, -8.999999999999992895, 3.374999999999999556 ) ) ;
#12265=COLOUR_RGB ( '',0.8941176470588234615, 0.8941176470588234615, 0.8941176470588234615 ) ;
#12286=CARTESIAN_POINT ( 'NONE',  ( 1.878215178125000939, -12.25316411605952283, 0.6281249993854848279 ) ) ;
#12290=CARTESIAN_POINT ( 'NONE',  ( -3.999999999999959144, -11.30940107675851891, 1.556249998770965925 ) ) ;
#12300=ORIENTED_EDGE ( 'NONE', *, *, #2589, .F. ) ;
#12310=CARTESIAN_POINT ( 'NONE',  ( 3.752267015613588906E-15, -4.381197846482986158, 2.756249998770968546 ) ) ;
#12314=CARTESIAN_POINT ( 'NONE',  ( 2.672651547586948120E-15, -13.33755215474602984, 2.840624999385484184 ) ) ;
#12318=EDGE_CURVE ( 'NONE', #20735, #19181, #24813, .T. ) ;
#12321=CARTESIAN_POINT ( 'NONE',  ( 3.735045420075836212E-15, -4.662447845253954171, 2.503124999385483385 ) ) ;
#12324=CARTESIAN_POINT ( 'NONE',  ( -3.756430356249996994, -8.999999999999992895, 1.828124999385484450 ) ) ;
#12329=ORIENTED_EDGE ( 'NONE', *, *, #1536, .T. ) ;
#12368=DIRECTION ( 'NONE',  ( 0.000000000000000000, 1.000000000000000000, 0.000000000000000000 ) ) ;
#12374=CARTESIAN_POINT ( 'NONE',  ( 3.756430356250003655, -8.999999999999992895, 4.640624999385483562 ) ) ;
#12389=CARTESIAN_POINT ( 'NONE',  ( 2.000000000000000888, -12.46410161513774817, 1.274999999999998357 ) ) ;
#12394=EDGE_CURVE ( 'NONE', #12847, #10226, #12118, .T. ) ;
#12400=ORIENTED_EDGE ( 'NONE', *, *, #10116, .T. ) ;
#12405=CARTESIAN_POINT ( 'NONE',  ( 3.735045420075836212E-15, -4.662447845253954171, 1.715624999385482852 ) ) ;
#12413=DIRECTION ( 'NONE',  ( -0.000000000000000000, -0.000000000000000000, -1.000000000000000000 ) ) ;
#12432=EDGE_LOOP ( 'NONE', ( #17043, #8611, #22469, #15637, #5207, #18205 ) ) ;
#12433=CARTESIAN_POINT ( 'NONE',  ( 3.469446951953614189E-15, -8.999999999999992895, 0.000000000000000000 ) ) ;
#12436=CARTESIAN_POINT ( 'NONE',  ( -3.756430356249995661, -6.831223922626973533, 1.790624999385484806 ) ) ;
#12439=DIRECTION ( 'NONE',  ( -0.000000000000000000, -0.000000000000000000, -1.000000000000000000 ) ) ;
#12443=CARTESIAN_POINT ( 'NONE',  ( 3.756430356250004099, -6.831223922626973533, 0.6281249993854786107 ) ) ;
#12444=CARTESIAN_POINT ( 'NONE',  ( -1.999999999999995781, -5.535898384862237620, 4.199999999999999289 ) ) ;
#12446=CARTESIAN_POINT ( 'NONE',  ( 3.756430356250003655, -8.999999999999992895, 1.603124999385485028 ) ) ;
#12480=EDGE_LOOP ( 'NONE', ( #927, #21185, #15465, #9827 ) ) ;
#12539=CARTESIAN_POINT ( 'NONE',  ( 1.878215178125004048, -5.746835883940462963, 1.678124999385483651 ) ) ;
#12544=CARTESIAN_POINT ( 'NONE',  ( 2.000000000000003997, -5.535898384862238508, 3.675000000000001155 ) ) ;
#12572=CARTESIAN_POINT ( 'NONE',  ( 3.735045420075836212E-15, -4.662447845253954171, 3.065624999385482052 ) ) ;
#12580=CARTESIAN_POINT ( 'NONE',  ( -3.756430356249995661, -6.831223922626973533, 2.128124999385482052 ) ) ;
#12582=CARTESIAN_POINT ( 'NONE',  ( 4.000000000000001776, -11.30940107675849760, 4.462500000000000355 ) ) ;
#12587=CARTESIAN_POINT ( 'NONE',  ( -1.878215178124995832, -5.746835883940462963, 2.203124999385484895 ) ) ;
#12615=ADVANCED_FACE ( 'NONE', ( #16484 ), #24446, .T. ) ;
#12626=CARTESIAN_POINT ( 'NONE',  ( 3.752267015613588906E-15, -4.381197846482986158, 1.462499999999998135 ) ) ;
#12631=ORIENTED_EDGE ( 'NONE', *, *, #18891, .F. ) ;
#12641=CARTESIAN_POINT ( 'NONE',  ( 2.672651547586948120E-15, -13.33755215474603162, 4.528124999385480187 ) ) ;
#12679=CARTESIAN_POINT ( 'NONE',  ( 3.756430356250002323, -11.16877607737301226, 2.465624999385482852 ) ) ;
#12697=DIRECTION ( 'NONE',  ( -0.000000000000000000, -0.000000000000000000, -1.000000000000000000 ) ) ;
#12698=CARTESIAN_POINT ( 'NONE',  ( 3.752267015613588906E-15, -4.381197846482986158, 3.656249998770967569 ) ) ;
#12701=ORIENTED_EDGE ( 'NONE', *, *, #1688, .F. ) ;
#12713=CARTESIAN_POINT ( 'NONE',  ( 3.735045420075836212E-15, -4.662447845253954171, 1.715624999385482852 ) ) ;
#12716=FACE_OUTER_BOUND ( 'NONE', #15275, .T. ) ;
#12718=CARTESIAN_POINT ( 'NONE',  ( 3.735045420075836212E-15, -4.662447845253954171, 2.953124999385479565 ) ) ;
#12720=CARTESIAN_POINT ( 'NONE',  ( 4.000000000000003553, -6.690598923241489970, 3.637499999999998845 ) ) ;
#12723=CARTESIAN_POINT ( 'NONE',  ( -3.756430356249997438, -11.16877607737301048, 2.315624999385482496 ) ) ;
#12724=DIRECTION ( 'NONE',  ( -0.000000000000000000, -0.000000000000000000, -1.000000000000000000 ) ) ;
#12752=DIRECTION ( 'NONE',  ( 1.000000000000000000, 0.000000000000000000, 0.000000000000000000 ) ) ;
#12755=CARTESIAN_POINT ( 'NONE',  ( 4.000000000000003553, -8.999999999999992895, 1.350000000000000533 ) ) ;
#12764=CARTESIAN_POINT ( 'NONE',  ( 2.000000000000000888, -12.46410161513774817, 4.368749998770966592 ) ) ;
#12774=CARTESIAN_POINT ( 'NONE',  ( -1.999999999999995781, -5.535898384862237620, 1.049999999999998934 ) ) ;
#12801=CARTESIAN_POINT ( 'NONE',  ( 4.000000000000003553, -8.999999999999992895, 1.799999999999999600 ) ) ;
#12802=CARTESIAN_POINT ( 'NONE',  ( 3.756430356250003655, -8.999999999999992895, 2.053124999385484095 ) ) ;
#12823=VERTEX_POINT ( 'NONE', #22194 ) ;
#12832=CARTESIAN_POINT ( 'NONE',  ( 3.756430356250002323, -11.16877607737301226, 4.715624999385485516 ) ) ;
#12834=EDGE_CURVE ( 'NONE', #7795, #13776, #13966, .T. ) ;
#12837=CARTESIAN_POINT ( 'NONE',  ( 1.878215178125000939, -12.25316411605952283, 4.115624999385482319 ) ) ;
#12843=CARTESIAN_POINT ( 'NONE',  ( -1.878215178124998497, -12.25316411605951927, 1.903124999385483296 ) ) ;
#12847=VERTEX_POINT ( 'NONE', #11980 ) ;
#12877=CARTESIAN_POINT ( 'NONE',  ( 2.672651547586948120E-15, -13.33755215474602984, 0.4781249993854826963 ) ) ;
#12878=ORIENTED_EDGE ( 'NONE', *, *, #19831, .T. ) ;
#12884=ORIENTED_EDGE ( 'NONE', *, *, #21494, .F. ) ;
#12929=CARTESIAN_POINT ( 'NONE',  ( -1.878215178124998497, -12.25316411605951927, 1.003124999385485161 ) ) ;
#12938=DIRECTION ( 'NONE',  ( -1.000000000000000000, 0.000000000000000000, 0.000000000000000000 ) ) ;
#12965=CARTESIAN_POINT ( 'NONE',  ( 3.756430356250003655, -8.999999999999992895, 0.1406249993854830072 ) ) ;
#12966=CARTESIAN_POINT ( 'NONE',  ( 2.000000000000003997, -5.535898384862238508, 0.4687499987709661808 ) ) ;
#12970=CARTESIAN_POINT ( 'NONE',  ( -1.878215178124998497, -12.25316411605951927, 4.490624999385482319 ) ) ;
#12977=CARTESIAN_POINT ( 'NONE',  ( 1.878215178125004048, -5.746835883940462963, 4.378124999385484273 ) ) ;
#13068=CARTESIAN_POINT ( 'NONE',  ( 3.756430356250002323, -11.16877607737301226, 3.815624999385482052 ) ) ;
#13078=LINE ( 'NONE', #22877, #3438 ) ;
#13093=VERTEX_POINT ( 'NONE', #4523 ) ;
#13101=CARTESIAN_POINT ( 'NONE',  ( -1.878215178124998497, -12.25316411605951927, 4.603124999385483918 ) ) ;
#13102=CARTESIAN_POINT ( 'NONE',  ( 3.752267015613588906E-15, -4.381197846482986158, 2.756249998770968102 ) ) ;
#13109=CARTESIAN_POINT ( 'NONE',  ( -3.756430356249995661, -6.831223922626973533, 3.028124999385485072 ) ) ;
#13113=CARTESIAN_POINT ( 'NONE',  ( 3.756430356250003655, -8.999999999999992895, 0.1968749993854837510 ) ) ;
#13114=CARTESIAN_POINT ( 'NONE',  ( -3.756430356249996994, -8.999999999999992895, 3.628124999385483829 ) ) ;
#13137=ADVANCED_FACE ( 'NONE', ( #13165 ), #15253, .T. ) ;
#13154=DIRECTION ( 'NONE',  ( -0.000000000000000000, -0.000000000000000000, -1.000000000000000000 ) ) ;
#13163=PRODUCT_CONTEXT ( 'NONE', #21129, 'mechanical' ) ;
#13165=FACE_OUTER_BOUND ( 'NONE', #1417, .T. ) ;
#13174=CARTESIAN_POINT ( 'NONE',  ( 4.000000000000003553, -8.999999999999992895, 1.350000000000000533 ) ) ;
#13190=CARTESIAN_POINT ( 'NONE',  ( -3.756430356249996994, -8.999999999999992895, 1.715624999385483074 ) ) ;
#13208=VERTEX_POINT ( 'NONE', #14990 ) ;
#13221=CARTESIAN_POINT ( 'NONE',  ( -1.878215178124995832, -5.746835883940462963, 4.003124999385484273 ) ) ;
#13222=CARTESIAN_POINT ( 'NONE',  ( 2.000000000000003997, -5.535898384862238508, 0.9187499987709686344 ) ) ;
#13223=DIRECTION ( 'NONE',  ( 1.000000000000000000, 0.000000000000000000, 0.000000000000000000 ) ) ;
#13227=CARTESIAN_POINT ( 'NONE',  ( -3.999999999999997335, -11.30940107675849404, 0.2624999999999988454 ) ) ;
#13236=CARTESIAN_POINT ( 'NONE',  ( -3.999999999999996447, -8.999999999999992895, 4.218749998770966236 ) ) ;
#13246=EDGE_CURVE ( 'NONE', #9331, #9030, #16639, .T. ) ;
#13282=CARTESIAN_POINT ( 'NONE',  ( 3.469446951953614189E-15, -8.999999999999992895, 18.00000000000000000 ) ) ;
#13313=CARTESIAN_POINT ( 'NONE',  ( 3.756430356250003655, -8.999999999999992895, 0.1406249993854830072 ) ) ;
#13315=AXIS2_PLACEMENT_3D ( 'NONE', #4357, #10111, #16530 ) ;
#13351=CARTESIAN_POINT ( 'NONE',  ( 1.878215178125000939, -12.25316411605952283, 0.9656249993854824076 ) ) ;
#13352=CARTESIAN_POINT ( 'NONE',  ( -1.999999999999995781, -5.535898384862237620, 1.893749998770968723 ) ) ;
#13353=CARTESIAN_POINT ( 'NONE',  ( 0.000000000000000000, 0.000000000000000000, 0.000000000000000000 ) ) ;
#13360=CARTESIAN_POINT ( 'NONE',  ( -1.999999999999998224, -12.46410161513774639, 1.649999999999998579 ) ) ;
#13363=CARTESIAN_POINT ( 'NONE',  ( -3.999999999999996447, -8.999999999999992895, 0.000000000000000000 ) ) ;
#13365=CARTESIAN_POINT ( 'NONE',  ( -1.878215178124998497, -12.25316411605951927, 3.253124999385483829 ) ) ;
#13371=EDGE_LOOP ( 'NONE', ( #14366, #19662, #861, #16893 ) ) ;
#13380=ADVANCED_FACE ( 'NONE', ( #24994 ), #18864, .T. ) ;
#13396=VERTEX_POINT ( 'NONE', #18986 ) ;
#13445=( BOUNDED_CURVE ( )  B_SPLINE_CURVE ( 2, ( #14900, #22481, #12544, #24960, #20375, #4562, #22352 ),
 .UNSPECIFIED., .F., .F. ) 
 B_SPLINE_CURVE_WITH_KNOTS ( ( 3, 2, 2, 3 ),
 ( 0.7999999999999999334, 0.8166666666666665408, 0.8333333333333332593, 0.8499999999999998668 ),
 .UNSPECIFIED. ) 
 CURVE ( )  GEOMETRIC_REPRESENTATION_ITEM ( )  RATIONAL_B_SPLINE_CURVE ( ( 1.000000000000000888, 0.8660254037844378194, 1.000000000000000000, 0.8660254037844387076, 1.000000000000000000, 0.8660254037844395958, 0.9999999999999991118 ) ) 
 REPRESENTATION_ITEM ( '' )  );
#13455=CARTESIAN_POINT ( 'NONE',  ( 1.878215178125004048, -5.746835883940462963, 1.565624999385482274 ) ) ;
#13457=CARTESIAN_POINT ( 'NONE',  ( -1.878215178124998497, -12.25316411605951927, 4.153124999385485516 ) ) ;
#13491=CARTESIAN_POINT ( 'NONE',  ( 3.756430356250003655, -8.999999999999992895, 2.840624999385484184 ) ) ;
#13492=CARTESIAN_POINT ( 'NONE',  ( 4.000000000000003553, -8.999999999999992895, 1.743749998770967924 ) ) ;
#13496=CARTESIAN_POINT ( 'NONE',  ( 2.620986760973688460E-15, -13.61880215351699874, 0.7875000000000005329 ) ) ;
#13501=CARTESIAN_POINT ( 'NONE',  ( -3.756430356249996105, -6.831223922626973533, 4.490624999385483207 ) ) ;
#13524=CYLINDRICAL_SURFACE ( 'NONE', #1285, 4.000000000000000000 ) ;
#13576=CARTESIAN_POINT ( 'NONE',  ( 3.735045420075836212E-15, -4.662447845253954171, 1.153124999385480409 ) ) ;
#13577=CARTESIAN_POINT ( 'NONE',  ( 3.756430356250002323, -11.16877607737301226, 4.715624999385485516 ) ) ;
#13583=CARTESIAN_POINT ( 'NONE',  ( 3.469446951953614189E-15, -8.999999999999992895, 18.00000000000000000 ) ) ;
#13590=CARTESIAN_POINT ( 'NONE',  ( 4.000000000000003553, -8.999999999999992895, 2.249999999999998668 ) ) ;
#13593=VERTEX_POINT ( 'NONE', #21849 ) ;
#13597=ORIENTED_EDGE ( 'NONE', *, *, #11664, .T. ) ;
#13602=EDGE_CURVE ( 'NONE', #12823, #1770, #1334, .T. ) ;
#13609=CARTESIAN_POINT ( 'NONE',  ( 3.756430356250003655, -8.999999999999992895, 1.940624999385482496 ) ) ;
#13610=CARTESIAN_POINT ( 'NONE',  ( 2.000000000000000888, -12.46410161513774817, 3.018749998770966503 ) ) ;
#13614=CARTESIAN_POINT ( 'NONE',  ( -3.999999999999996003, -6.690598923241487306, 2.887499999999999289 ) ) ;
#13622=LINE ( 'NONE', #21589, #1197 ) ;
#13624=ORIENTED_EDGE ( 'NONE', *, *, #8861, .F. ) ;
#13672=CARTESIAN_POINT ( 'NONE',  ( -4.000000000000057732, -6.690598923241522833, 4.631249998770965881 ) ) ;
#13684=ORIENTED_EDGE ( 'NONE', *, *, #18697, .T. ) ;
#13691=CARTESIAN_POINT ( 'NONE',  ( 3.756430356250003211, -6.831223922626973533, 2.428124999385481431 ) ) ;
#13711=CARTESIAN_POINT ( 'NONE',  ( 2.620986760973688460E-15, -13.61880215351699874, 2.587499999999999467 ) ) ;
#13725=CARTESIAN_POINT ( 'NONE',  ( -1.878215178124995832, -5.746835883940462963, 2.090624999385483296 ) ) ;
#13726=CARTESIAN_POINT ( 'NONE',  ( -3.756430356249995661, -6.831223922626973533, 0.4406249993854817193 ) ) ;
#13735=CARTESIAN_POINT ( 'NONE',  ( 2.000000000000003997, -5.535898384862238508, 0.9750000000000001998 ) ) ;
#13738=CARTESIAN_POINT ( 'NONE',  ( 2.620986760973688460E-15, -13.61880215351699874, 2.531249998770966236 ) ) ;
#13762=CARTESIAN_POINT ( 'NONE',  ( -2.999999999999996891, -8.999999999999992895, 0.000000000000000000 ) ) ;
#13771=CARTESIAN_POINT ( 'NONE',  ( -1.878215178124998497, -12.25316411605951927, 0.5531249993854860936 ) ) ;
#13776=VERTEX_POINT ( 'NONE', #12158 ) ;
#13777=ORIENTED_EDGE ( 'NONE', *, *, #5528, .F. ) ;
#13812=ORIENTED_EDGE ( 'NONE', *, *, #19418, .F. ) ;
#13828=CARTESIAN_POINT ( 'NONE',  ( 3.756430356250003655, -8.999999999999992895, 4.190624999385480720 ) ) ;
#13837=DIRECTION ( 'NONE',  ( -1.000000000000000000, 0.000000000000000000, 0.000000000000000000 ) ) ;
#13866=CARTESIAN_POINT ( 'NONE',  ( 3.735045420075836212E-15, -4.662447845253954171, 3.853124999385482585 ) ) ;
#13867=CARTESIAN_POINT ( 'NONE',  ( 4.000000000000003553, -6.690598923241489970, 4.031249998770966236 ) ) ;
#13873=CARTESIAN_POINT ( 'NONE',  ( -3.999999999999997335, -11.30940107675849404, 2.062499999999998224 ) ) ;
#13885=LINE ( 'NONE', #1978, #16276 ) ;
#13894=ORIENTED_EDGE ( 'NONE', *, *, #11086, .F. ) ;
#13910=CARTESIAN_POINT ( 'NONE',  ( 3.756430356250003211, -6.831223922626973533, 0.2906249993854817526 ) ) ;
#13946=EDGE_LOOP ( 'NONE', ( #6702, #21693, #23466, #7061 ) ) ;
#13948=EDGE_CURVE ( 'NONE', #6968, #18161, #1155, .T. ) ;
#13961=CARTESIAN_POINT ( 'NONE',  ( 1.878215178125000939, -12.25316411605952283, 4.115624999385482319 ) ) ;
#13964=ADVANCED_FACE ( 'NONE', ( #15171 ), #25097, .T. ) ;
#13966=( BOUNDED_CURVE ( )  B_SPLINE_CURVE ( 2, ( #7809, #1932, #4013, #2059, #19832, #2196, #8325 ),
 .UNSPECIFIED., .F., .F. ) 
 B_SPLINE_CURVE_WITH_KNOTS ( ( 3, 2, 2, 3 ),
 ( 0.8499999999999998668, 0.8666666666666664742, 0.8833333333333330817, 0.8999999999999996891 ),
 .UNSPECIFIED. ) 
 CURVE ( )  GEOMETRIC_REPRESENTATION_ITEM ( )  RATIONAL_B_SPLINE_CURVE ( ( 1.000000000000000888, 0.8660254037844378194, 1.000000000000000000, 0.8660254037844387076, 1.000000000000000000, 0.8660254037844413721, 0.9999999999999973355 ) ) 
 REPRESENTATION_ITEM ( '' )  );
#13993=CARTESIAN_POINT ( 'NONE',  ( 3.735045420075836212E-15, -4.662447845253954171, 3.403124999385483296 ) ) ;
#13994=CARTESIAN_POINT ( 'NONE',  ( 3.752267015613588906E-15, -4.381197846482986158, 3.656249998770967569 ) ) ;
#14003=DIRECTION ( 'NONE',  ( 1.000000000000000000, 0.000000000000000000, 0.000000000000000000 ) ) ;
#14011=CARTESIAN_POINT ( 'NONE',  ( 4.000000000000003553, -8.999999999999992895, 1.799999999999999600 ) ) ;
#14020=ORIENTED_EDGE ( 'NONE', *, *, #3778, .T. ) ;
#14059=CARTESIAN_POINT ( 'NONE',  ( -3.999999999999982681, -6.690598923241479312, 0.1875000000000006384 ) ) ;
#14071=DIRECTION ( 'NONE',  ( -0.000000000000000000, -0.000000000000000000, -1.000000000000000000 ) ) ;
#14083=CARTESIAN_POINT ( 'NONE',  ( -3.756430356249996994, -8.999999999999992895, 3.065624999385483385 ) ) ;
#14102=CARTESIAN_POINT ( 'NONE',  ( -3.999999999999966249, -11.30940107675851181, 2.962499999999997691 ) ) ;
#14115=( BOUNDED_CURVE ( )  B_SPLINE_CURVE ( 2, ( #15551, #22058, #15934, #21939, #23765, #17639, #5720 ),
 .UNSPECIFIED., .F., .F. ) 
 B_SPLINE_CURVE_WITH_KNOTS ( ( 3, 2, 2, 3 ),
 ( 0.3500000000000000888, 0.3666666666666666963, 0.3833333333333333592, 0.3999999999999999667 ),
 .UNSPECIFIED. ) 
 CURVE ( )  GEOMETRIC_REPRESENTATION_ITEM ( )  RATIONAL_B_SPLINE_CURVE ( ( 0.9999999999999991118, 0.8660254037844395958, 1.000000000000000000, 0.8660254037844387076, 1.000000000000000000, 0.8660254037844391517, 0.9999999999999995559 ) ) 
 REPRESENTATION_ITEM ( '' )  );
#14120=CARTESIAN_POINT ( 'NONE',  ( 3.756430356250002323, -11.16877607737301226, 4.603124999385482141 ) ) ;
#14121=CARTESIAN_POINT ( 'NONE',  ( -1.878215178124995832, -5.746835883940462963, 0.4031249993854852942 ) ) ;
#14132=AXIS2_PLACEMENT_3D ( 'NONE', #14688, #2518, #10225 ) ;
#14152=CARTESIAN_POINT ( 'NONE',  ( -3.756430356249995661, -6.831223922626973533, 3.590624999385483740 ) ) ;
#14159=CARTESIAN_POINT ( 'NONE',  ( 3.756430356250003655, -8.999999999999992895, 1.490624999385483429 ) ) ;
#14162=CARTESIAN_POINT ( 'NONE',  ( 3.735045420075836212E-15, -4.662447845253954171, 0.3656249993854837621 ) ) ;
#14174=ORIENTED_EDGE ( 'NONE', *, *, #12318, .T. ) ;
#14204=ORIENTED_EDGE ( 'NONE', *, *, #19020, .T. ) ;
#14217=CARTESIAN_POINT ( 'NONE',  ( -3.756430356249997438, -11.16877607737301048, 2.653124999385483296 ) ) ;
#14218=ADVANCED_FACE ( 'NONE', ( #20345 ), #12123, .T. ) ;
#14245=ORIENTED_EDGE ( 'NONE', *, *, #21962, .F. ) ;
#14259=CARTESIAN_POINT ( 'NONE',  ( 2.620986760973688460E-15, -13.61880215351699874, 4.331249998770966059 ) ) ;
#14267=CARTESIAN_POINT ( 'NONE',  ( 3.878215178125003604, -8.999999999999992895, 0.07031249969274150358 ) ) ;
#14278=LINE ( 'NONE', #20389, #5824 ) ;
#14281=( BOUNDED_CURVE ( )  B_SPLINE_CURVE ( 2, ( #9748, #5688, #21779, #20060, #5815, #24115, #6199 ),
 .UNSPECIFIED., .F., .F. ) 
 B_SPLINE_CURVE_WITH_KNOTS ( ( 3, 2, 2, 3 ),
 ( 0.1499999999999996891, 0.1666666666666665741, 0.1833333333333334592, 0.2000000000000003719 ),
 .UNSPECIFIED. ) 
 CURVE ( )  GEOMETRIC_REPRESENTATION_ITEM ( )  RATIONAL_B_SPLINE_CURVE ( ( 1.000000000000002665, 0.8660254037844363761, 1.000000000000000000, 0.8660254037844387076, 1.000000000000000000, 0.8660254037844358210, 1.000000000000002887 ) ) 
 REPRESENTATION_ITEM ( '' )  );
#14284=ADVANCED_FACE ( 'NONE', ( #9899 ), #17885, .T. ) ;
#14285=EDGE_LOOP ( 'NONE', ( #21888, #1558, #11289, #20820 ) ) ;
#14294=CARTESIAN_POINT ( 'NONE',  ( -3.756430356249997882, -11.16877607737301226, 3.215624999385481964 ) ) ;
#14300=DIRECTION ( 'NONE',  ( 1.000000000000000000, 0.000000000000000000, -0.000000000000000000 ) ) ;
#14301=CARTESIAN_POINT ( 'NONE',  ( -1.878215178124998497, -12.25316411605951927, 2.240624999385484095 ) ) ;
#14306=CARTESIAN_POINT ( 'NONE',  ( 3.756430356250002323, -11.16877607737301403, 1.115624999385483429 ) ) ;
#14357=CARTESIAN_POINT ( 'NONE',  ( -1.999999999999995781, -5.535898384862237620, 3.300000000000000711 ) ) ;
#14366=ORIENTED_EDGE ( 'NONE', *, *, #1536, .F. ) ;
#14391=CARTESIAN_POINT ( 'NONE',  ( -3.756430356249997882, -11.16877607737301226, 2.315624999385482496 ) ) ;
#14419=CARTESIAN_POINT ( 'NONE',  ( -1.878215178124998497, -12.25316411605951927, 3.703124999385482674 ) ) ;
#14423=CARTESIAN_POINT ( 'NONE',  ( -3.756430356249996994, -8.999999999999992895, 2.165624999385482141 ) ) ;
#14424=CARTESIAN_POINT ( 'NONE',  ( 4.000000000000003553, -8.999999999999992895, 4.500000000000000888 ) ) ;
#14427=CARTESIAN_POINT ( 'NONE',  ( -1.878215178124995832, -5.746835883940462963, 3.103124999385483029 ) ) ;
#14430=ORIENTED_EDGE ( 'NONE', *, *, #10638, .T. ) ;
#14491=CARTESIAN_POINT ( 'NONE',  ( -3.999999999999996447, -8.999999999999992895, 18.00000000000000000 ) ) ;
#14494=CARTESIAN_POINT ( 'NONE',  ( 4.000000000000003553, -8.999999999999992895, 18.00000000000000000 ) ) ;
#14505=CARTESIAN_POINT ( 'NONE',  ( 3.756430356250002323, -11.16877607737301226, 1.115624999385483429 ) ) ;
#14534=CARTESIAN_POINT ( 'NONE',  ( 3.756430356250002323, -11.16877607737301226, 2.915624999385482141 ) ) ;
#14537=CYLINDRICAL_SURFACE ( 'NONE', #15501, 4.000000000000000000 ) ;
#14539=CIRCLE ( 'NONE', #8268, 3.000000000000000444 ) ;
#14540=CARTESIAN_POINT ( 'NONE',  ( 2.672651547586948120E-15, -13.33755215474602984, 1.378124999385482274 ) ) ;
#14542=CARTESIAN_POINT ( 'NONE',  ( 4.000000000000001776, -11.30940107675849760, 4.012499999999996625 ) ) ;
#14545=CARTESIAN_POINT ( 'NONE',  ( -3.756430356249996994, -8.999999999999992895, 1.378124999385485605 ) ) ;
#14547=AXIS2_PLACEMENT_3D ( 'NONE', #14267, #3932, #14003 ) ;
#14560=AXIS2_PLACEMENT_3D ( 'NONE', #16180, #20225, #13837 ) ;
#14612=LINE ( 'NONE', #24812, #19258 ) ;
#14634=CARTESIAN_POINT ( 'NONE',  ( -3.999999999999966249, -11.30940107675851181, 3.356249998770968190 ) ) ;
#14637=CARTESIAN_POINT ( 'NONE',  ( -1.878215178124998497, -12.25316411605951927, 2.353124999385485694 ) ) ;
#14655=EDGE_LOOP ( 'NONE', ( #2426, #23908, #17810, #16082 ) ) ;
#14671=CARTESIAN_POINT ( 'NONE',  ( 1.878215178125004048, -5.746835883940462963, 2.128124999385486049 ) ) ;
#14679=CARTESIAN_POINT ( 'NONE',  ( 3.756430356250002323, -11.16877607737301226, 1.453124999385484228 ) ) ;
#14681=CARTESIAN_POINT ( 'NONE',  ( 2.000000000000000888, -12.46410161513774817, 3.075000000000001510 ) ) ;
#14686=CARTESIAN_POINT ( 'NONE',  ( 3.756430356250002323, -11.16877607737301403, 2.915624999385482141 ) ) ;
#14688=CARTESIAN_POINT ( 'NONE',  ( 3.469446951953614189E-15, -8.999999999999992895, 18.00000000000000000 ) ) ;
#14726=CARTESIAN_POINT ( 'NONE',  ( -1.878215178124998497, -12.25316411605951927, 0.4406249993854846614 ) ) ;
#14731=CARTESIAN_POINT ( 'NONE',  ( -4.000000000000012434, -11.30940107675848516, 4.256249998770963217 ) ) ;
#14773=CARTESIAN_POINT ( 'NONE',  ( 2.672651547586948120E-15, -13.33755215474602984, 2.840624999385484184 ) ) ;
#14802=CARTESIAN_POINT ( 'NONE',  ( -2.999999999999996891, -8.999999999999992895, 18.00000000000000000 ) ) ;
#14805=CARTESIAN_POINT ( 'NONE',  ( 1.878215178125004048, -5.746835883940462963, 0.6656249993854841396 ) ) ;
#14806=CARTESIAN_POINT ( 'NONE',  ( 3.752267015613588906E-15, -4.381197846482986158, 0.5062499987709696558 ) ) ;
#14811=CARTESIAN_POINT ( 'NONE',  ( 3.735045420075836212E-15, -4.662447845253954171, 3.853124999385482585 ) ) ;
#14813=CARTESIAN_POINT ( 'NONE',  ( 4.000000000000003553, -8.999999999999992895, 3.149999999999999911 ) ) ;
#14817=CARTESIAN_POINT ( 'NONE',  ( 3.756430356250003655, -8.999999999999992895, 2.053124999385484095 ) ) ;
#14830=EDGE_CURVE ( 'NONE', #7795, #4035, #9655, .T. ) ;
#14845=CARTESIAN_POINT ( 'NONE',  ( -1.999999999999995781, -5.535898384862237620, 3.243749998770965703 ) ) ;
#14852=CARTESIAN_POINT ( 'NONE',  ( 3.756430356250003655, -8.999999999999992895, 0.1406249993854830072 ) ) ;
#14864=CARTESIAN_POINT ( 'NONE',  ( 2.672651547586948120E-15, -13.33755215474602984, 4.528124999385480187 ) ) ;
#14884=VERTEX_POINT ( 'NONE', #16062 ) ;
#14894=CARTESIAN_POINT ( 'NONE',  ( 3.756430356250003655, -8.999999999999992895, 1.603124999385485028 ) ) ;
#14899=CARTESIAN_POINT ( 'NONE',  ( -4.000000000000010658, -6.690598923241495299, 1.931249998770966814 ) ) ;
#14900=CARTESIAN_POINT ( 'NONE',  ( 4.000000000000003553, -8.999999999999992895, 3.599999999999999201 ) ) ;
#14927=CARTESIAN_POINT ( 'NONE',  ( 3.756430356250004099, -6.831223922626973533, 0.1781249993854828739 ) ) ;
#14931=CARTESIAN_POINT ( 'NONE',  ( -3.999999999999996447, -8.999999999999992895, 0.6749999999999984901 ) ) ;
#14932=CARTESIAN_POINT ( 'NONE',  ( -1.999999999999995781, -5.535898384862237620, 0.1500000000000008271 ) ) ;
#14935=CARTESIAN_POINT ( 'NONE',  ( 3.752267015613588906E-15, -4.381197846482986158, 3.712500000000000355 ) ) ;
#14937=CARTESIAN_POINT ( 'NONE',  ( -3.756430356249997438, -11.16877607737301048, 3.215624999385481964 ) ) ;
#14957=DIRECTION ( 'NONE',  ( -1.000000000000000000, 0.000000000000000000, 0.000000000000000000 ) ) ;
#14990=CARTESIAN_POINT ( 'NONE',  ( -3.999999999999996447, -8.999999999999992895, 2.418749998770966414 ) ) ;
#15021=CARTESIAN_POINT ( 'NONE',  ( -1.878215178124995832, -5.746835883940462963, 1.190624999385481830 ) ) ;
#15023=CARTESIAN_POINT ( 'NONE',  ( 3.756430356250003655, -8.999999999999992895, 3.403124999385484628 ) ) ;
#15062=CARTESIAN_POINT ( 'NONE',  ( -1.878215178124995832, -5.746835883940462963, 1.190624999385481830 ) ) ;
#15063=CARTESIAN_POINT ( 'NONE',  ( -1.999999999999995781, -5.535898384862237620, 2.343749998770968013 ) ) ;
#15068=CIRCLE ( 'NONE', #18393, 4.000000000000000000 ) ;
#15069=CARTESIAN_POINT ( 'NONE',  ( -1.878215178124995832, -5.746835883940462963, 3.440624999385483829 ) ) ;
#15074=CARTESIAN_POINT ( 'NONE',  ( 3.756430356250003655, -8.999999999999992895, 3.853124999385483473 ) ) ;
#15124=( BOUNDED_SURFACE ( )  B_SPLINE_SURFACE ( 1, 2, ( 
 ( #9717, #3956, #21607, #1875, #9836, #17701, #10090, #17819, #15731, #25784, #7869, #18090, #7487, #3685, #11665, #5916, #15476, #3565, #21874, #11538, #23827, #19891, #1990, #8012, #17564, #36, #15997, #7624, #19505, #25669, #23694, #9958, #23964, #4206, #24214, #428, #24352, #4740, #4461, #12713, #6301, #12436, #6681, #12185, #24082, #20403, #10472, #2258, #18473, #8532, #14671, #8396, #16119, #10214, #22652, #20552, #561, #24594, #18212, #20680, #16386, #2506, #6164, #2379, #4593, #16513, #293, #8263, #24475, #12314, #6552, #14534, #8142, #22511, #20158, #12572, #2644, #10605, #18595, #14294, #20282, #22259, #2763, #4340, #10333, #682, #16242, #18329, #10724, #14152, #6432, #8649, #14419, #16628, #171, #22120, #22377, #8780, #2889, #7332, #13221, #19097, #17288, #20806, #15312, #18980, #21075, #16769, #20946, #23162, #1181, #10858, #18854, #9161, #4985, #25122, #13101, #801, #3152, #12832, #17151 ),
 ( #12965, #14927, #21327, #6948, #16903, #7210, #945, #8923, #25253, #24738, #22779, #1065, #23280, #24867, #14805, #15192, #22899, #24986, #3031, #6823, #5362, #5242, #13351, #9038, #7071, #17021, #4856, #11000, #15062, #3405, #23037, #5125, #11118, #18710, #19223, #21191, #3268, #11243, #1323, #9303, #5882, #17404, #21966, #3536, #25369, #23931, #17529, #17911, #13609, #7837, #1572, #5744, #13725, #21574, #6013, #21706, #19607, #3791, #15701, #9924, #11383, #9543, #25503, #9807, #19358, #1453, #25755, #2, #11768, #25637, #23793, #11893, #13491, #3922, #19862, #11507, #9424, #19478, #7977, #19746, #9683, #15440, #7592, #11630, #17669, #15963, #23667, #13993, #15577, #1845, #7453, #23413, #5498, #17789, #21459, #15821, #23545, #1960, #5628, #13866, #21841, #3653, #1710, #7718, #18780, #2348, #2091, #6135, #8850, #18057, #8114, #6398, #2227, #16088, #24051, #141, #10785, #14864, #20250, #14120, #4042 ) ),
 .UNSPECIFIED., .F., .F., .F. ) 
 B_SPLINE_SURFACE_WITH_KNOTS ( ( 2, 2 ),
 ( 3, 2, 2, 2, 2, 2, 2, 2, 2, 2, 2, 2, 2, 2, 2, 2, 2, 2, 2, 2, 2, 2, 2, 2, 2, 2, 2, 2, 2, 2, 2, 2, 2, 2, 2, 2, 2, 2, 2, 2, 2, 2, 2, 2, 2, 2, 2, 2, 2, 2, 2, 2, 2, 2, 2, 2, 2, 2, 2, 2, 3 ),
 ( 0.000000000000000000, 1.000000000000000000 ),
 ( 0.000000000000000000, 0.01666666666666666644, 0.03333333333333333287, 0.05000000000000000278, 0.06666666666666666574, 0.08333333333333332871, 0.1000000000000000056, 0.1166666666666666685, 0.1333333333333333315, 0.1499999999999999944, 0.1666666666666666574, 0.1833333333333333204, 0.2000000000000000111, 0.2166666666666666741, 0.2333333333333333370, 0.2500000000000000000, 0.2666666666666666630, 0.2833333333333333259, 0.2999999999999999889, 0.3166666666666666519, 0.3333333333333333148, 0.3499999999999999778, 0.3666666666666666408, 0.3833333333333333592, 0.4000000000000000222, 0.4166666666666666852, 0.4333333333333333481, 0.4500000000000000111, 0.4666666666666666741, 0.4833333333333333370, 0.5000000000000000000, 0.5166666666666667185, 0.5333333333333333259, 0.5500000000000000444, 0.5666666666666666519, 0.5833333333333333703, 0.5999999999999999778, 0.6166666666666666963, 0.6333333333333333037, 0.6500000000000000222, 0.6666666666666666297, 0.6833333333333333481, 0.6999999999999999556, 0.7166666666666666741, 0.7333333333333332815, 0.7500000000000000000, 0.7666666666666667185, 0.7833333333333333259, 0.8000000000000000444, 0.8166666666666666519, 0.8333333333333333703, 0.8499999999999999778, 0.8666666666666666963, 0.8833333333333333037, 0.9000000000000000222, 0.9166666666666666297, 0.9333333333333333481, 0.9499999999999999556, 0.9666666666666666741, 0.9833333333333332815, 1.000000000000000000 ),
 .UNSPECIFIED. ) 
 GEOMETRIC_REPRESENTATION_ITEM ( )  RATIONAL_B_SPLINE_SURFACE ( (
 ( 1.000000000000000000, 0.8660254037844387076, 1.000000000000000000, 0.8660254037844387076, 1.000000000000000000, 0.8660254037844387076, 1.000000000000000000, 0.8660254037844387076, 1.000000000000000000, 0.8660254037844387076, 1.000000000000000000, 0.8660254037844387076, 1.000000000000000000, 0.8660254037844387076, 1.000000000000000000, 0.8660254037844387076, 1.000000000000000000, 0.8660254037844387076, 1.000000000000000000, 0.8660254037844387076, 1.000000000000000000, 0.8660254037844387076, 1.000000000000000000, 0.8660254037844387076, 1.000000000000000000, 0.8660254037844387076, 1.000000000000000000, 0.8660254037844387076, 1.000000000000000000, 0.8660254037844387076, 1.000000000000000000, 0.8660254037844387076, 1.000000000000000000, 0.8660254037844387076, 1.000000000000000000, 0.8660254037844387076, 1.000000000000000000, 0.8660254037844387076, 1.000000000000000000, 0.8660254037844387076, 1.000000000000000000, 0.8660254037844387076, 1.000000000000000000, 0.8660254037844387076, 1.000000000000000000, 0.8660254037844387076, 1.000000000000000000, 0.8660254037844387076, 1.000000000000000000, 0.8660254037844387076, 1.000000000000000000, 0.8660254037844387076, 1.000000000000000000, 0.8660254037844387076, 1.000000000000000000, 0.8660254037844387076, 1.000000000000000000, 0.8660254037844387076, 1.000000000000000000, 0.8660254037844387076, 1.000000000000000000, 0.8660254037844387076, 1.000000000000000000, 0.8660254037844387076, 1.000000000000000000, 0.8660254037844387076, 1.000000000000000000, 0.8660254037844387076, 1.000000000000000000, 0.8660254037844387076, 1.000000000000000000, 0.8660254037844387076, 1.000000000000000000, 0.8660254037844387076, 1.000000000000000000, 0.8660254037844387076, 1.000000000000000000, 0.8660254037844387076, 1.000000000000000000, 0.8660254037844387076, 1.000000000000000000, 0.8660254037844387076, 1.000000000000000000, 0.8660254037844387076, 1.000000000000000000, 0.8660254037844387076, 1.000000000000000000, 0.8660254037844387076, 1.000000000000000000, 0.8660254037844387076, 1.000000000000000000, 0.8660254037844387076, 1.000000000000000000, 0.8660254037844387076, 1.000000000000000000, 0.8660254037844387076, 1.000000000000000000, 0.8660254037844387076, 1.000000000000000000, 0.8660254037844387076, 1.000000000000000000, 0.8660254037844387076, 1.000000000000000000, 0.8660254037844387076, 1.000000000000000000, 0.8660254037844387076, 1.000000000000000000, 0.8660254037844387076, 1.000000000000000000, 0.8660254037844387076, 1.000000000000000000, 0.8660254037844387076, 1.000000000000000000, 0.8660254037844387076, 1.000000000000000000, 0.8660254037844387076, 1.000000000000000000, 0.8660254037844387076, 1.000000000000000000, 0.8660254037844387076, 1.000000000000000000),
 ( 1.000000000000000000, 0.8660254037844387076, 1.000000000000000000, 0.8660254037844387076, 1.000000000000000000, 0.8660254037844387076, 1.000000000000000000, 0.8660254037844387076, 1.000000000000000000, 0.8660254037844387076, 1.000000000000000000, 0.8660254037844387076, 1.000000000000000000, 0.8660254037844387076, 1.000000000000000000, 0.8660254037844387076, 1.000000000000000000, 0.8660254037844387076, 1.000000000000000000, 0.8660254037844387076, 1.000000000000000000, 0.8660254037844387076, 1.000000000000000000, 0.8660254037844387076, 1.000000000000000000, 0.8660254037844387076, 1.000000000000000000, 0.8660254037844387076, 1.000000000000000000, 0.8660254037844387076, 1.000000000000000000, 0.8660254037844387076, 1.000000000000000000, 0.8660254037844387076, 1.000000000000000000, 0.8660254037844387076, 1.000000000000000000, 0.8660254037844387076, 1.000000000000000000, 0.8660254037844387076, 1.000000000000000000, 0.8660254037844387076, 1.000000000000000000, 0.8660254037844387076, 1.000000000000000000, 0.8660254037844387076, 1.000000000000000000, 0.8660254037844387076, 1.000000000000000000, 0.8660254037844387076, 1.000000000000000000, 0.8660254037844387076, 1.000000000000000000, 0.8660254037844387076, 1.000000000000000000, 0.8660254037844387076, 1.000000000000000000, 0.8660254037844387076, 1.000000000000000000, 0.8660254037844387076, 1.000000000000000000, 0.8660254037844387076, 1.000000000000000000, 0.8660254037844387076, 1.000000000000000000, 0.8660254037844387076, 1.000000000000000000, 0.8660254037844387076, 1.000000000000000000, 0.8660254037844387076, 1.000000000000000000, 0.8660254037844387076, 1.000000000000000000, 0.8660254037844387076, 1.000000000000000000, 0.8660254037844387076, 1.000000000000000000, 0.8660254037844387076, 1.000000000000000000, 0.8660254037844387076, 1.000000000000000000, 0.8660254037844387076, 1.000000000000000000, 0.8660254037844387076, 1.000000000000000000, 0.8660254037844387076, 1.000000000000000000, 0.8660254037844387076, 1.000000000000000000, 0.8660254037844387076, 1.000000000000000000, 0.8660254037844387076, 1.000000000000000000, 0.8660254037844387076, 1.000000000000000000, 0.8660254037844387076, 1.000000000000000000, 0.8660254037844387076, 1.000000000000000000, 0.8660254037844387076, 1.000000000000000000, 0.8660254037844387076, 1.000000000000000000, 0.8660254037844387076, 1.000000000000000000, 0.8660254037844387076, 1.000000000000000000, 0.8660254037844387076, 1.000000000000000000, 0.8660254037844387076, 1.000000000000000000, 0.8660254037844387076, 1.000000000000000000, 0.8660254037844387076, 1.000000000000000000, 0.8660254037844387076, 1.000000000000000000, 0.8660254037844387076, 1.000000000000000000, 0.8660254037844387076, 1.000000000000000000) ) ) 
 REPRESENTATION_ITEM ( '' )  SURFACE ( )  );
#15158=ORIENTED_EDGE ( 'NONE', *, *, #19418, .T. ) ;
#15162=CARTESIAN_POINT ( 'NONE',  ( 3.756430356250002323, -11.16877607737301403, 1.453124999385484228 ) ) ;
#15165=CARTESIAN_POINT ( 'NONE',  ( 3.756430356250002323, -11.16877607737301226, 4.265624999385481786 ) ) ;
#15166=( NAMED_UNIT ( * ) SI_UNIT ( $, .STERADIAN. ) SOLID_ANGLE_UNIT ( ) );
#15171=FACE_OUTER_BOUND ( 'NONE', #19562, .T. ) ;
#15188=ORIENTED_EDGE ( 'NONE', *, *, #22869, .F. ) ;
#15192=CARTESIAN_POINT ( 'NONE',  ( 3.735045420075836212E-15, -4.662447845253954171, 0.7031249993854805647 ) ) ;
#15193=CARTESIAN_POINT ( 'NONE',  ( -3.999999999999996003, -6.690598923241487306, 2.381249998770966769 ) ) ;
#15199=CARTESIAN_POINT ( 'NONE',  ( 2.000000000000003997, -5.535898384862238508, 0.5250000000000011324 ) ) ;
#15205=CARTESIAN_POINT ( 'NONE',  ( -1.999999999999995781, -5.535898384862237620, 0.5437499987709683014 ) ) ;
#15207=CARTESIAN_POINT ( 'NONE',  ( 2.000000000000003997, -5.535898384862238508, 4.068749998770968546 ) ) ;
#15232=VERTEX_POINT ( 'NONE', #25548 ) ;
#15253=CYLINDRICAL_SURFACE ( 'NONE', #11673, 4.000000000000000000 ) ;
#15275=EDGE_LOOP ( 'NONE', ( #6737, #4413, #24495, #4512 ) ) ;
#15281=CARTESIAN_POINT ( 'NONE',  ( -3.756430356249996994, -8.999999999999992895, 4.528124999385485516 ) ) ;
#15294=CARTESIAN_POINT ( 'NONE',  ( 2.000000000000000888, -12.46410161513774817, 4.424999999999998046 ) ) ;
#15309=DIRECTION ( 'NONE',  ( -0.000000000000000000, -0.000000000000000000, -1.000000000000000000 ) ) ;
#15312=CARTESIAN_POINT ( 'NONE',  ( -1.878215178124998497, -12.25316411605951927, 4.153124999385485516 ) ) ;
#15313=CARTESIAN_POINT ( 'NONE',  ( 2.620986760973688460E-15, -13.61880215351699874, 2.081249998770966947 ) ) ;
#15317=CARTESIAN_POINT ( 'NONE',  ( 4.000000000000001776, -11.30940107675849760, 0.8624999999999984901 ) ) ;
#15334=ORIENTED_EDGE ( 'NONE', *, *, #12318, .F. ) ;
#15400=CARTESIAN_POINT ( 'NONE',  ( 3.756430356250003211, -6.831223922626973533, 0.6281249993854786107 ) ) ;
#15408=EDGE_CURVE ( 'NONE', #16617, #21696, #14539, .T. ) ;
#15416=ORIENTED_EDGE ( 'NONE', *, *, #19096, .T. ) ;
#15440=CARTESIAN_POINT ( 'NONE',  ( 2.672651547586948120E-15, -13.33755215474602984, 3.178124999385481431 ) ) ;
#15441=CARTESIAN_POINT ( 'NONE',  ( 4.000000000000003553, -6.690598923241489970, 0.8812499987709634386 ) ) ;
#15442=ADVANCED_FACE ( 'NONE', ( #2270 ), #6444, .T. ) ;
#15446=CARTESIAN_POINT ( 'NONE',  ( 4.000000000000003553, -8.999999999999992895, 3.993749998770966592 ) ) ;
#15449=CARTESIAN_POINT ( 'NONE',  ( -1.999999999999998224, -12.46410161513774639, 1.199999999999999734 ) ) ;
#15455=ADVANCED_FACE ( 'NONE', ( #574 ), #20693, .T. ) ;
#15456=CARTESIAN_POINT ( 'NONE',  ( -3.756430356249996994, -8.999999999999992895, 4.528124999385485516 ) ) ;
#15459=CARTESIAN_POINT ( 'NONE',  ( 3.469446951953614189E-15, -8.999999999999992895, 18.00000000000000000 ) ) ;
#15465=ORIENTED_EDGE ( 'NONE', *, *, #7804, .T. ) ;
#15476=CARTESIAN_POINT ( 'NONE',  ( -1.878215178124995832, -5.746835883940462963, 0.8531249993854843616 ) ) ;
#15501=AXIS2_PLACEMENT_3D ( 'NONE', #4211, #12439, #22656 ) ;
#15539=( LENGTH_UNIT ( ) NAMED_UNIT ( * ) SI_UNIT ( .MILLI., .METRE. ) );
#15542=CARTESIAN_POINT ( 'NONE',  ( -3.756430356249996994, -8.999999999999992895, 1.265624999385484006 ) ) ;
#15544=CARTESIAN_POINT ( 'NONE',  ( 1.878215178125004048, -5.746835883940462963, 3.928124999385485872 ) ) ;
#15551=CARTESIAN_POINT ( 'NONE',  ( -3.999999999999996447, -8.999999999999992895, 1.968749998770967569 ) ) ;
#15560=CARTESIAN_POINT ( 'NONE',  ( 3.000000000000003997, -8.999999999999992895, 0.000000000000000000 ) ) ;
#15577=CARTESIAN_POINT ( 'NONE',  ( -1.878215178124995832, -5.746835883940462963, 3.440624999385483829 ) ) ;
#15578=CARTESIAN_POINT ( 'NONE',  ( 4.000000000000003553, -8.999999999999992895, 1.293749998770969079 ) ) ;
#15582=CARTESIAN_POINT ( 'NONE',  ( -3.999999999999996447, -8.999999999999992895, 3.768749998770966947 ) ) ;
#15584=CARTESIAN_POINT ( 'NONE',  ( 2.620986760973688460E-15, -13.61880215351699874, 2.587499999999999467 ) ) ;
#15600=EDGE_CURVE ( 'NONE', #9331, #7533, #3667, .T. ) ;
#15619=STYLED_ITEM ( 'NONE', ( #16057 ), #5978 ) ;
#15632=CARTESIAN_POINT ( 'NONE',  ( 4.000000000000003553, -8.999999999999992895, 4.049999999999998046 ) ) ;
#15637=ORIENTED_EDGE ( 'NONE', *, *, #2589, .T. ) ;
#15668=CARTESIAN_POINT ( 'NONE',  ( -3.756430356249997438, -11.16877607737301048, 2.203124999385479565 ) ) ;
#15701=CARTESIAN_POINT ( 'NONE',  ( 1.878215178125000939, -12.25316411605952283, 2.315624999385482941 ) ) ;
#15702=CARTESIAN_POINT ( 'NONE',  ( -3.999999999999996003, -6.690598923241487306, 4.631249998770964993 ) ) ;
#15703=DIRECTION ( 'NONE',  ( 0.000000000000000000, 0.000000000000000000, 1.000000000000000000 ) ) ;
#15708=CARTESIAN_POINT ( 'NONE',  ( 2.620986760973688460E-15, -13.61880215351699874, 1.237499999999996270 ) ) ;
#15731=CARTESIAN_POINT ( 'NONE',  ( -1.878215178124998497, -12.25316411605951927, 0.5531249993854860936 ) ) ;
#15742=ORIENTED_EDGE ( 'NONE', *, *, #13602, .F. ) ;
#15783=CARTESIAN_POINT ( 'NONE',  ( -3.756430356249997438, -11.16877607737301048, 3.103124999385483029 ) ) ;
#15802=CARTESIAN_POINT ( 'NONE',  ( 2.000000000000003997, -5.535898384862238508, 2.325000000000000622 ) ) ;
#15821=CARTESIAN_POINT ( 'NONE',  ( 3.756430356250002323, -11.16877607737301226, 3.703124999385482674 ) ) ;
#15822=CARTESIAN_POINT ( 'NONE',  ( -3.999999999999996447, -8.999999999999992895, 3.768749998770966947 ) ) ;
#15827=CARTESIAN_POINT ( 'NONE',  ( 2.000000000000000888, -12.46410161513774817, 0.8249999999999992895 ) ) ;
#15866=CARTESIAN_POINT ( 'NONE',  ( 3.756430356250003655, -8.999999999999992895, 0.2531249993854844949 ) ) ;
#15910=VERTEX_POINT ( 'NONE', #2623 ) ;
#15923=CARTESIAN_POINT ( 'NONE',  ( 3.756430356250003655, -8.999999999999992895, 2.390624999385481342 ) ) ;
#15934=CARTESIAN_POINT ( 'NONE',  ( -1.999999999999998224, -12.46410161513774639, 2.043749998770966414 ) ) ;
#15959=EDGE_CURVE ( 'NONE', #24155, #17175, #11442, .T. ) ;
#15963=CARTESIAN_POINT ( 'NONE',  ( 3.756430356250004099, -6.831223922626973533, 3.328124999385480898 ) ) ;
#15964=CARTESIAN_POINT ( 'NONE',  ( 4.000000000000003553, -8.999999999999992895, 4.893749998770967835 ) ) ;
#15971=CARTESIAN_POINT ( 'NONE',  ( 4.000000000000003553, -8.999999999999992895, 0.9000000000000014655 ) ) ;
#15997=CARTESIAN_POINT ( 'NONE',  ( 1.878215178125004048, -5.746835883940462963, 1.228124999385484584 ) ) ;
#15998=CARTESIAN_POINT ( 'NONE',  ( 2.000000000000003997, -5.535898384862238508, 1.368749998770967702 ) ) ;
#16055=CARTESIAN_POINT ( 'NONE',  ( -3.756430356249996105, -6.831223922626973533, 3.478124999385480809 ) ) ;
#16057=PRESENTATION_STYLE_ASSIGNMENT (( #20090 ) ) ;
#16062=CARTESIAN_POINT ( 'NONE',  ( -3.999999999999996447, -8.999999999999992895, 4.275000000000001243 ) ) ;
#16067=ORIENTED_EDGE ( 'NONE', *, *, #2225, .T. ) ;
#16074=CARTESIAN_POINT ( 'NONE',  ( 3.469446951953614189E-15, -8.999999999999992895, 18.00000000000000000 ) ) ;
#16082=ORIENTED_EDGE ( 'NONE', *, *, #16724, .F. ) ;
#16088=CARTESIAN_POINT ( 'NONE',  ( -3.756430356249995661, -6.831223922626973533, 4.378124999385480720 ) ) ;
#16089=CARTESIAN_POINT ( 'NONE',  ( 3.756430356250003655, -8.999999999999992895, 0.2531249993854844949 ) ) ;
#16092=CARTESIAN_POINT ( 'NONE',  ( -4.000000000000039968, -11.30940107675846740, 0.7124999999999979128 ) ) ;
#16108=( BOUNDED_CURVE ( )  B_SPLINE_CURVE ( 2, ( #2545, #12226, #6202, #10515, #22556, #8683, #24636 ),
 .UNSPECIFIED., .F., .F. ) 
 B_SPLINE_CURVE_WITH_KNOTS ( ( 3, 2, 2, 3 ),
 ( 0.4499999999999998446, 0.4666666666666665075, 0.4833333333333331150, 0.4999999999999997780 ),
 .UNSPECIFIED. ) 
 CURVE ( )  GEOMETRIC_REPRESENTATION_ITEM ( )  RATIONAL_B_SPLINE_CURVE ( ( 1.000000000000001332, 0.8660254037844373753, 1.000000000000000000, 0.8660254037844387076, 1.000000000000000000, 0.8660254037844404840, 0.9999999999999982236 ) ) 
 REPRESENTATION_ITEM ( '' )  );
#16119=CARTESIAN_POINT ( 'NONE',  ( -1.878215178124995832, -5.746835883940462963, 2.203124999385484895 ) ) ;
#16126=CARTESIAN_POINT ( 'NONE',  ( 2.672651547586948120E-15, -13.33755215474602984, 0.9281249993854824298 ) ) ;
#16141=CARTESIAN_POINT ( 'NONE',  ( -3.999999999999973355, -6.690598923241474871, 2.381249998770965881 ) ) ;
#16173=CARTESIAN_POINT ( 'NONE',  ( -3.756430356249997438, -11.16877607737301048, 3.553124999385482763 ) ) ;
#16180=CARTESIAN_POINT ( 'NONE',  ( 3.469446951953614189E-15, -8.999999999999992895, 18.00000000000000000 ) ) ;
#16211=CARTESIAN_POINT ( 'NONE',  ( -3.756430356249996994, -8.999999999999992895, 0.4781249993854840286 ) ) ;
#16214=CARTESIAN_POINT ( 'NONE',  ( -3.999999999999996447, -8.999999999999992895, 1.518749998770968501 ) ) ;
#16221=CARTESIAN_POINT ( 'NONE',  ( 2.000000000000003997, -5.535898384862238508, 2.774999999999999467 ) ) ;
#16237=EDGE_CURVE ( 'NONE', #18161, #20603, #9907, .T. ) ;
#16242=CARTESIAN_POINT ( 'NONE',  ( 1.878215178125004048, -5.746835883940462963, 3.478124999385483029 ) ) ;
#16251=CARTESIAN_POINT ( 'NONE',  ( 2.672651547586948120E-15, -13.33755215474602984, 1.828124999385481786 ) ) ;
#16252=CARTESIAN_POINT ( 'NONE',  ( 4.000000000000003553, -8.999999999999992895, 1.293749998770969079 ) ) ;
#16254=CARTESIAN_POINT ( 'NONE',  ( -3.756430356249996994, -8.999999999999992895, 3.178124999385484983 ) ) ;
#16263=PLANE ( 'NONE',  #13315 ) ;
#16267=VECTOR ( 'NONE', #18362, 1000.000000000000000 ) ;
#16276=VECTOR ( 'NONE', #1861, 1000.000000000000000 ) ;
#16278=LINE ( 'NONE', #4102, #16267 ) ;
#16297=ORIENTED_EDGE ( 'NONE', *, *, #18847, .F. ) ;
#16302=FACE_OUTER_BOUND ( 'NONE', #14285, .T. ) ;
#16336=EDGE_LOOP ( 'NONE', ( #8348, #3194, #4033, #9799 ) ) ;
#16350=CARTESIAN_POINT ( 'NONE',  ( 3.735045420075836212E-15, -4.662447845253954171, 3.065624999385482052 ) ) ;
#16353=EDGE_CURVE ( 'NONE', #12823, #5385, #24651, .T. ) ;
#16380=CARTESIAN_POINT ( 'NONE',  ( -3.999999999999949818, -6.690598923241462437, 2.831249998770965615 ) ) ;
#16383=DIRECTION ( 'NONE',  ( -0.000000000000000000, -0.000000000000000000, 1.000000000000000000 ) ) ;
#16385=VECTOR ( 'NONE', #19482, 1000.000000000000000 ) ;
#16386=CARTESIAN_POINT ( 'NONE',  ( 3.756430356250003655, -8.999999999999992895, 2.503124999385482941 ) ) ;
#16392=CARTESIAN_POINT ( 'NONE',  ( -3.756430356249997882, -11.16877607737301226, 1.753124999385479832 ) ) ;
#16393=CARTESIAN_POINT ( 'NONE',  ( 2.000000000000000888, -12.46410161513774817, 3.525000000000000355 ) ) ;
#16396=CARTESIAN_POINT ( 'NONE',  ( -3.756430356249996994, -8.999999999999992895, 2.728124999385482585 ) ) ;
#16423=( BOUNDED_CURVE ( )  B_SPLINE_CURVE ( 2, ( #15632, #1502, #23599, #3849, #11827, #1772, #9474 ),
 .UNSPECIFIED., .F., .F. ) 
 B_SPLINE_CURVE_WITH_KNOTS ( ( 3, 2, 2, 3 ),
 ( 0.8999999999999996891, 0.9166666666666665186, 0.9333333333333335702, 0.9500000000000003997 ),
 .UNSPECIFIED. ) 
 CURVE ( )  GEOMETRIC_REPRESENTATION_ITEM ( )  RATIONAL_B_SPLINE_CURVE ( ( 1.000000000000002665, 0.8660254037844360431, 1.000000000000000000, 0.8660254037844387076, 1.000000000000000000, 0.8660254037844351549, 1.000000000000003553 ) ) 
 REPRESENTATION_ITEM ( '' )  );
#16463=ORIENTED_EDGE ( 'NONE', *, *, #5556, .F. ) ;
#16478=VERTEX_POINT ( 'NONE', #13174 ) ;
#16481=LINE ( 'NONE', #22747, #8927 ) ;
#16482=CARTESIAN_POINT ( 'NONE',  ( -3.756430356249996994, -8.999999999999992895, 2.278124999385483740 ) ) ;
#16484=FACE_OUTER_BOUND ( 'NONE', #21318, .T. ) ;
#16491=CARTESIAN_POINT ( 'NONE',  ( 3.752267015613588906E-15, -4.381197846482986158, 0.9562499987709653926 ) ) ;
#16513=CARTESIAN_POINT ( 'NONE',  ( -3.756430356249995661, -6.831223922626973533, 2.690624999385480276 ) ) ;
#16514=CARTESIAN_POINT ( 'NONE',  ( -3.999999999999997335, -11.30940107675849404, 0.6562499987709655702 ) ) ;
#16519=CARTESIAN_POINT ( 'NONE',  ( 2.672651547586948120E-15, -13.33755215474602984, 2.728124999385481253 ) ) ;
#16521=CARTESIAN_POINT ( 'NONE',  ( 2.000000000000003997, -5.535898384862238508, 4.125000000000000000 ) ) ;
#16524=CARTESIAN_POINT ( 'NONE',  ( 1.878215178125000939, -12.25316411605952283, 1.528124999385482852 ) ) ;
#16530=DIRECTION ( 'NONE',  ( 1.000000000000000000, 0.000000000000000000, -0.000000000000000000 ) ) ;
#16532=CARTESIAN_POINT ( 'NONE',  ( -3.999999999999996447, -8.999999999999992895, 2.418749998770966414 ) ) ;
#16553=CARTESIAN_POINT ( 'NONE',  ( -3.999999999999996447, -8.999999999999992895, 1.574999999999999956 ) ) ;
#16599=CARTESIAN_POINT ( 'NONE',  ( 3.756430356250002323, -11.16877607737301226, 2.015624999385483118 ) ) ;
#16607=CARTESIAN_POINT ( 'NONE',  ( -3.999999999999996447, -8.999999999999992895, 1.068749998770966103 ) ) ;
#16617=VERTEX_POINT ( 'NONE', #20756 ) ;
#16628=CARTESIAN_POINT ( 'NONE',  ( 2.672651547586948120E-15, -13.33755215474602984, 3.740624999385483651 ) ) ;
#16634=CARTESIAN_POINT ( 'NONE',  ( -3.756430356249995661, -6.831223922626973533, 1.228124999385478144 ) ) ;
#16636=CARTESIAN_POINT ( 'NONE',  ( -3.999999999999996003, -6.690598923241487306, 3.337499999999999023 ) ) ;
#16639=( BOUNDED_CURVE ( )  B_SPLINE_CURVE ( 2, ( #11702, #5813, #7906, #5953, #17728, #14059, #6560 ),
 .UNSPECIFIED., .F., .F. ) 
 B_SPLINE_CURVE_WITH_KNOTS ( ( 3, 2, 2, 3 ),
 ( 0.000000000000000000, 0.01666666666666663521, 0.03333333333333327042, 0.04999999999999990563 ),
 .UNSPECIFIED. ) 
 CURVE ( )  GEOMETRIC_REPRESENTATION_ITEM ( )  RATIONAL_B_SPLINE_CURVE ( ( 1.000000000000000000, 0.8660254037844387076, 1.000000000000000000, 0.8660254037844387076, 1.000000000000000000, 0.8660254037844394848, 0.9999999999999992228 ) ) 
 REPRESENTATION_ITEM ( '' )  );
#16640=CARTESIAN_POINT ( 'NONE',  ( 3.756430356250003655, -8.999999999999992895, 1.153124999385485960 ) ) ;
#16641=DIRECTION ( 'NONE',  ( 1.000000000000000000, 0.000000000000000000, 0.000000000000000000 ) ) ;
#16659=AXIS2_PLACEMENT_3D ( 'NONE', #3946, #19769, #1864 ) ;
#16678=LINE ( 'NONE', #6087, #2104 ) ;
#16679=EDGE_CURVE ( 'NONE', #10674, #23645, #10275, .T. ) ;
#16684=CARTESIAN_POINT ( 'NONE',  ( -3.999999999999996447, -8.999999999999992895, 0.6187499987709670357 ) ) ;
#16704=CARTESIAN_POINT ( 'NONE',  ( 3.469446951953614189E-15, -8.999999999999992895, 18.00000000000000000 ) ) ;
#16724=EDGE_CURVE ( 'NONE', #12847, #337, #17473, .T. ) ;
#16728=CARTESIAN_POINT ( 'NONE',  ( 4.000000000000003553, -8.999999999999992895, 3.543749998770967302 ) ) ;
#16732=CARTESIAN_POINT ( 'NONE',  ( 3.756430356250003655, -8.999999999999992895, 1.153124999385485960 ) ) ;
#16741=DIRECTION ( 'NONE',  ( 0.000000000000000000, 0.000000000000000000, 1.000000000000000000 ) ) ;
#16769=CARTESIAN_POINT ( 'NONE',  ( 3.756430356250002323, -11.16877607737301226, 4.265624999385481786 ) ) ;
#16770=CARTESIAN_POINT ( 'NONE',  ( 4.000000000000003553, -8.999999999999992895, 0.3937499987709675020 ) ) ;
#16776=CARTESIAN_POINT ( 'NONE',  ( 3.756430356250002323, -11.16877607737301226, 3.253124999385482941 ) ) ;
#16778=CARTESIAN_POINT ( 'NONE',  ( 3.752267015613588906E-15, -4.381197846482986158, 4.162500000000000533 ) ) ;
#16782=CARTESIAN_POINT ( 'NONE',  ( 3.735045420075836212E-15, -4.662447845253954171, 2.165624999385483029 ) ) ;
#16786=ORIENTED_EDGE ( 'NONE', *, *, #16353, .T. ) ;
#16801=( BOUNDED_CURVE ( )  B_SPLINE_CURVE ( 2, ( #12755, #8572, #18249, #12626, #6346, #10521, #16553 ),
 .UNSPECIFIED., .F., .F. ) 
 B_SPLINE_CURVE_WITH_KNOTS ( ( 3, 2, 2, 3 ),
 ( 0.3000000000000002109, 0.3166666666666668184, 0.3333333333333334814, 0.3500000000000000888 ),
 .UNSPECIFIED. ) 
 CURVE ( )  GEOMETRIC_REPRESENTATION_ITEM ( )  RATIONAL_B_SPLINE_CURVE ( ( 0.9999999999999982236, 0.8660254037844404840, 1.000000000000000000, 0.8660254037844387076, 1.000000000000000000, 0.8660254037844378194, 1.000000000000000888 ) ) 
 REPRESENTATION_ITEM ( '' )  );
#16812=VECTOR ( 'NONE', #12413, 1000.000000000000000 ) ;
#16816=DIRECTION ( 'NONE',  ( -0.000000000000000000, -0.000000000000000000, -1.000000000000000000 ) ) ;
#16849=DIRECTION ( 'NONE',  ( -0.000000000000000000, -0.000000000000000000, -1.000000000000000000 ) ) ;
#16854=ORIENTED_EDGE ( 'NONE', *, *, #466, .F. ) ;
#16870=CARTESIAN_POINT ( 'NONE',  ( -1.878215178124995832, -5.746835883940462963, 2.203124999385484895 ) ) ;
#16875=EDGE_CURVE ( 'NONE', #18617, #20603, #5284, .T. ) ;
#16893=ORIENTED_EDGE ( 'NONE', *, *, #5528, .T. ) ;
#16903=CARTESIAN_POINT ( 'NONE',  ( -1.878215178124995832, -5.746835883940462963, 0.2906249993854838065 ) ) ;
#16909=CARTESIAN_POINT ( 'NONE',  ( 3.756430356250004099, -6.831223922626973533, 3.328124999385480898 ) ) ;
#16913=CARTESIAN_POINT ( 'NONE',  ( -3.999999999999996447, -8.999999999999992895, 2.868749998770965703 ) ) ;
#16914=CARTESIAN_POINT ( 'NONE',  ( 3.756430356250002323, -11.16877607737301403, 3.815624999385481164 ) ) ;
#16972=EDGE_CURVE ( 'NONE', #17764, #4035, #7925, .T. ) ;
#17021=CARTESIAN_POINT ( 'NONE',  ( 3.756430356250004099, -6.831223922626973533, 1.078124999385482452 ) ) ;
#17026=CARTESIAN_POINT ( 'NONE',  ( 3.756430356250002323, -11.16877607737301226, 4.153124999385482852 ) ) ;
#17031=CARTESIAN_POINT ( 'NONE',  ( -3.756430356249997438, -11.16877607737301048, 4.565624999385485161 ) ) ;
#17043=ORIENTED_EDGE ( 'NONE', *, *, #19273, .F. ) ;
#17065=CARTESIAN_POINT ( 'NONE',  ( -3.756430356249996994, -8.999999999999992895, 0.3656249993854825409 ) ) ;
#17082=AXIS2_PLACEMENT_3D ( 'NONE', #25858, #8331, #7946 ) ;
#17114=CARTESIAN_POINT ( 'NONE',  ( 1.878215178125004048, -5.746835883940462963, 1.115624999385483207 ) ) ;
#17116=CARTESIAN_POINT ( 'NONE',  ( 1.878215178125004048, -5.746835883940462963, 4.378124999385484273 ) ) ;
#17117=( NAMED_UNIT ( * ) PLANE_ANGLE_UNIT ( ) SI_UNIT ( $, .RADIAN. ) );
#17134=CARTESIAN_POINT ( 'NONE',  ( -3.999999999999996447, -8.999999999999992895, 4.275000000000001243 ) ) ;
#17151=CARTESIAN_POINT ( 'NONE',  ( 3.756430356250003655, -8.999999999999992895, 4.753124999385485161 ) ) ;
#17152=CARTESIAN_POINT ( 'NONE',  ( 4.000000000000003553, -6.690598923241489970, 1.331249998770967169 ) ) ;
#17159=CARTESIAN_POINT ( 'NONE',  ( 2.000000000000003997, -5.535898384862238508, 0.07499999999999867883 ) ) ;
#17166=CARTESIAN_POINT ( 'NONE',  ( 4.000000000000003553, -6.690598923241489970, 0.4312499987709677018 ) ) ;
#17169=CARTESIAN_POINT ( 'NONE',  ( -3.999999999999980904, -6.690598923241480200, 4.181249998770965703 ) ) ;
#17175=VERTEX_POINT ( 'NONE', #22886 ) ;
#17176=CARTESIAN_POINT ( 'NONE',  ( 4.000000000000003553, -8.999999999999992895, 4.893749998770967835 ) ) ;
#17181=ORIENTED_EDGE ( 'NONE', *, *, #3339, .T. ) ;
#17254=CARTESIAN_POINT ( 'NONE',  ( -1.878215178124998497, -12.25316411605951927, 1.340624999385482630 ) ) ;
#17268=( BOUNDED_CURVE ( )  B_SPLINE_CURVE ( 2, ( #8150, #7878, #24091, #25675, #20167, #6174, #12053 ),
 .UNSPECIFIED., .F., .F. ) 
 B_SPLINE_CURVE_WITH_KNOTS ( ( 3, 2, 2, 3 ),
 ( 0.7500000000000000000, 0.7666666666666667185, 0.7833333333333332149, 0.7999999999999999334 ),
 .UNSPECIFIED. ) 
 CURVE ( )  GEOMETRIC_REPRESENTATION_ITEM ( )  RATIONAL_B_SPLINE_CURVE ( ( 1.000000000000000000, 0.8660254037844387076, 1.000000000000000000, 0.8660254037844387076, 1.000000000000000000, 0.8660254037844395958, 0.9999999999999991118 ) ) 
 REPRESENTATION_ITEM ( '' )  );
#17285=CARTESIAN_POINT ( 'NONE',  ( 4.000000000000003553, -8.999999999999992895, 3.599999999999999201 ) ) ;
#17288=CARTESIAN_POINT ( 'NONE',  ( -3.756430356249996994, -8.999999999999992895, 4.078124999385482674 ) ) ;
#17289=CARTESIAN_POINT ( 'NONE',  ( 2.620986760973688460E-15, -13.61880215351699874, 0.7312499987709674132 ) ) ;
#17293=CARTESIAN_POINT ( 'NONE',  ( -3.756430356249996994, -8.999999999999992895, 3.965624999385481519 ) ) ;
#17298=CARTESIAN_POINT ( 'NONE',  ( 3.756430356250003655, -8.999999999999992895, 4.303124999385482319 ) ) ;
#17357=CARTESIAN_POINT ( 'NONE',  ( -3.999999999999996447, -8.999999999999992895, 18.00000000000000000 ) ) ;
#17376=CARTESIAN_POINT ( 'NONE',  ( -3.756430356249995661, -6.831223922626973533, 4.040624999385483918 ) ) ;
#17377=CARTESIAN_POINT ( 'NONE',  ( 3.469446951953614189E-15, -8.999999999999992895, 18.00000000000000000 ) ) ;
#17404=CARTESIAN_POINT ( 'NONE',  ( -3.756430356249995661, -6.831223922626973533, 1.678124999385481875 ) ) ;
#17405=CARTESIAN_POINT ( 'NONE',  ( -3.999999999999996447, -8.999999999999992895, 2.418749998770966414 ) ) ;
#17410=CARTESIAN_POINT ( 'NONE',  ( -3.999999999999997335, -11.30940107675849404, 3.806249998770963927 ) ) ;
#17411=LINE ( 'NONE', #7458, #16385 ) ;
#17412=CARTESIAN_POINT ( 'NONE',  ( -3.999999999999997335, -11.30940107675849404, 2.512500000000001510 ) ) ;
#17417=CARTESIAN_POINT ( 'NONE',  ( 3.756430356250002323, -11.16877607737301403, 4.265624999385481786 ) ) ;
#17451=VECTOR ( 'NONE', #25608, 1000.000000000000000 ) ;
#17473=LINE ( 'NONE', #17357, #19157 ) ;
#17489=CARTESIAN_POINT ( 'NONE',  ( -1.878215178124998497, -12.25316411605951927, 0.4406249993854846614 ) ) ;
#17492=CARTESIAN_POINT ( 'NONE',  ( -1.878215178124998497, -12.25316411605951927, 3.703124999385482674 ) ) ;
#17515=EDGE_CURVE ( 'NONE', #15910, #23645, #12136, .T. ) ;
#17529=CARTESIAN_POINT ( 'NONE',  ( 1.878215178125000939, -12.25316411605952283, 1.865624999385483873 ) ) ;
#17530=CARTESIAN_POINT ( 'NONE',  ( 3.752267015613588906E-15, -4.381197846482986158, 2.306249998770968368 ) ) ;
#17538=CARTESIAN_POINT ( 'NONE',  ( -3.999999999999996447, -8.999999999999992895, 2.024999999999999023 ) ) ;
#17563=AXIS2_PLACEMENT_3D ( 'NONE', #4387, #12368, #18258 ) ;
#17564=CARTESIAN_POINT ( 'NONE',  ( 3.756430356250003655, -8.999999999999992895, 1.153124999385485960 ) ) ;
#17620=ORIENTED_EDGE ( 'NONE', *, *, #19831, .F. ) ;
#17622=( NAMED_UNIT ( * ) SI_UNIT ( $, .STERADIAN. ) SOLID_ANGLE_UNIT ( ) );
#17626=CARTESIAN_POINT ( 'NONE',  ( 1.878215178125000939, -12.25316411605952283, 0.9656249993854824076 ) ) ;
#17639=CARTESIAN_POINT ( 'NONE',  ( 3.999999999999994227, -11.30940107675849937, 2.156249998770968457 ) ) ;
#17659=PRODUCT_DEFINITION ( 'UNKNOWN', '', #7286, #24842 ) ;
#17663=MECHANICAL_DESIGN_GEOMETRIC_PRESENTATION_REPRESENTATION('',(#20584),#7629);
#17669=CARTESIAN_POINT ( 'NONE',  ( 3.756430356250003655, -8.999999999999992895, 3.290624999385483029 ) ) ;
#17670=CARTESIAN_POINT ( 'NONE',  ( 4.000000000000003553, -6.690598923241489970, 2.681249998770966592 ) ) ;
#17675=CARTESIAN_POINT ( 'NONE',  ( -3.999999999999997335, -11.30940107675849404, 1.612499999999998046 ) ) ;
#17677=CARTESIAN_POINT ( 'NONE',  ( -3.999999999999996447, -8.999999999999992895, 2.418749998770966414 ) ) ;
#17685=EDGE_LOOP ( 'NONE', ( #4849, #5259, #677, #10462 ) ) ;
#17692=ORIENTED_EDGE ( 'NONE', *, *, #22750, .T. ) ;
#17701=CARTESIAN_POINT ( 'NONE',  ( -3.756430356249995661, -6.831223922626973533, 0.4406249993854817193 ) ) ;
#17707=CARTESIAN_POINT ( 'NONE',  ( 1.878215178125004048, -5.746835883940462963, 0.3281249993854831737 ) ) ;
#17728=CARTESIAN_POINT ( 'NONE',  ( -1.999999999999995781, -5.535898384862237620, 0.1500000000000008271 ) ) ;
#17751=CARTESIAN_POINT ( 'NONE',  ( 3.756430356250002323, -11.16877607737301403, 3.703124999385482674 ) ) ;
#17764=VERTEX_POINT ( 'NONE', #5074 ) ;
#17768=DIRECTION ( 'NONE',  ( 0.8660254037844397068, -0.000000000000000000, 0.4999999999999983347 ) ) ;
#17783=( BOUNDED_CURVE ( )  B_SPLINE_CURVE ( 2, ( #25383, #21340, #2799, #7731, #14845, #10765, #9438 ),
 .UNSPECIFIED., .F., .F. ) 
 B_SPLINE_CURVE_WITH_KNOTS ( ( 3, 2, 2, 3 ),
 ( 0.6000000000000004219, 0.6166666666666670293, 0.6333333333333336368, 0.6500000000000002442 ),
 .UNSPECIFIED. ) 
 CURVE ( )  GEOMETRIC_REPRESENTATION_ITEM ( )  RATIONAL_B_SPLINE_CURVE ( ( 0.9999999999999964473, 0.8660254037844422603, 1.000000000000000000, 0.8660254037844387076, 1.000000000000000000, 0.8660254037844369313, 1.000000000000001776 ) ) 
 REPRESENTATION_ITEM ( '' )  );
#17788=( BOUNDED_CURVE ( )  B_SPLINE_CURVE ( 2, ( #24061, #4567, #4717, #16491, #4440, #2620, #16607 ),
 .UNSPECIFIED., .F., .F. ) 
 B_SPLINE_CURVE_WITH_KNOTS ( ( 3, 2, 2, 3 ),
 ( 0.09999999999999981126, 0.1166666666666664326, 0.1333333333333330539, 0.1499999999999996891 ),
 .UNSPECIFIED. ) 
 CURVE ( )  GEOMETRIC_REPRESENTATION_ITEM ( )  RATIONAL_B_SPLINE_CURVE ( ( 1.000000000000001776, 0.8660254037844372643, 1.000000000000000000, 0.8660254037844387076, 1.000000000000000000, 0.8660254037844411501, 0.9999999999999975575 ) ) 
 REPRESENTATION_ITEM ( '' )  );
#17789=CARTESIAN_POINT ( 'NONE',  ( 2.672651547586948120E-15, -13.33755215474602984, 3.628124999385485161 ) ) ;
#17790=CARTESIAN_POINT ( 'NONE',  ( -1.999999999999998224, -12.46410161513774639, 3.393749998770966503 ) ) ;
#17796=CARTESIAN_POINT ( 'NONE',  ( 3.752267015613588906E-15, -4.381197846482986158, 1.912500000000001865 ) ) ;
#17810=ORIENTED_EDGE ( 'NONE', *, *, #3893, .T. ) ;
#17816=ORIENTED_EDGE ( 'NONE', *, *, #16875, .F. ) ;
#17819=CARTESIAN_POINT ( 'NONE',  ( -3.756430356249997882, -11.16877607737301226, 0.5156249993854836733 ) ) ;
#17878=CARTESIAN_POINT ( 'NONE',  ( -1.878215178124995832, -5.746835883940462963, 4.340624999385481964 ) ) ;
#17885=CYLINDRICAL_SURFACE ( 'NONE', #17082, 4.000000000000000000 ) ;
#17911=CARTESIAN_POINT ( 'NONE',  ( 3.756430356250002323, -11.16877607737301226, 1.903124999385483740 ) ) ;
#17912=CARTESIAN_POINT ( 'NONE',  ( -3.999999999999996447, -8.999999999999992895, 4.668749998770968190 ) ) ;
#17916=CARTESIAN_POINT ( 'NONE',  ( 2.620986760973688460E-15, -13.61880215351699874, 0.7875000000000005329 ) ) ;
#17917=CARTESIAN_POINT ( 'NONE',  ( -3.999999999999996003, -6.690598923241487306, 2.437499999999999556 ) ) ;
#17943=ADVANCED_FACE ( 'NONE', ( #22567 ), #22978, .T. ) ;
#17949=AXIS2_PLACEMENT_3D ( 'NONE', #6977, #1091, #14957 ) ;
#17964=ORIENTED_EDGE ( 'NONE', *, *, #8390, .T. ) ;
#18012=ORIENTED_EDGE ( 'NONE', *, *, #21494, .T. ) ;
#18016=CARTESIAN_POINT ( 'NONE',  ( -1.878215178124998497, -12.25316411605951927, 2.690624999385483385 ) ) ;
#18057=CARTESIAN_POINT ( 'NONE',  ( 3.756430356250004099, -6.831223922626973533, 4.228124999385484806 ) ) ;
#18058=CARTESIAN_POINT ( 'NONE',  ( 4.000000000000003553, -8.999999999999992895, 4.443749998770965881 ) ) ;
#18090=CARTESIAN_POINT ( 'NONE',  ( 3.756430356250002323, -11.16877607737301226, 0.6656249993854835845 ) ) ;
#18098=CARTESIAN_POINT ( 'NONE',  ( 3.756430356250003655, -8.999999999999992895, 1.040624999385484584 ) ) ;
#18106=ORIENTED_EDGE ( 'NONE', *, *, #16972, .F. ) ;
#18146=EDGE_CURVE ( 'NONE', #22527, #3646, #11127, .T. ) ;
#18153=CARTESIAN_POINT ( 'NONE',  ( 3.756430356250002323, -11.16877607737301403, 2.353124999385479477 ) ) ;
#18159=DIRECTION ( 'NONE',  ( -0.000000000000000000, -0.000000000000000000, -1.000000000000000000 ) ) ;
#18161=VERTEX_POINT ( 'NONE', #19105 ) ;
#18176=ADVANCED_FACE ( 'NONE', ( #9551 ), #10193, .F. ) ;
#18183=CARTESIAN_POINT ( 'NONE',  ( 4.000000000000003553, -6.690598923241489970, 3.581249998770965615 ) ) ;
#18192=DIRECTION ( 'NONE',  ( 1.000000000000000000, 0.000000000000000000, 0.000000000000000000 ) ) ;
#18194=CARTESIAN_POINT ( 'NONE',  ( 2.000000000000000888, -12.46410161513774817, 1.725000000000000755 ) ) ;
#18205=ORIENTED_EDGE ( 'NONE', *, *, #6163, .F. ) ;
#18212=CARTESIAN_POINT ( 'NONE',  ( 1.878215178125000939, -12.25316411605952283, 2.428124999385484539 ) ) ;
#18216=DIRECTION ( 'NONE',  ( 0.000000000000000000, 0.000000000000000000, 1.000000000000000000 ) ) ;
#18217=CARTESIAN_POINT ( 'NONE',  ( 1.878215178125004048, -5.746835883940462963, 0.6656249993854841396 ) ) ;
#18220=LINE ( 'NONE', #7755, #5870 ) ;
#18222=DIRECTION ( 'NONE',  ( -1.000000000000000000, 0.000000000000000000, 0.000000000000000000 ) ) ;
#18226=ORIENTED_EDGE ( 'NONE', *, *, #5566, .F. ) ;
#18249=CARTESIAN_POINT ( 'NONE',  ( 2.000000000000003997, -5.535898384862238508, 1.424999999999999156 ) ) ;
#18258=DIRECTION ( 'NONE',  ( -1.000000000000000000, 0.000000000000000000, 0.000000000000000000 ) ) ;
#18289=ORIENTED_EDGE ( 'NONE', *, *, #14830, .F. ) ;
#18295=AXIS2_PLACEMENT_3D ( 'NONE', #6566, #12724, #18222 ) ;
#18299=CARTESIAN_POINT ( 'NONE',  ( -1.999999999999998224, -12.46410161513774639, 4.743749998770967480 ) ) ;
#18300=EDGE_CURVE ( 'NONE', #13208, #25772, #19599, .T. ) ;
#18311=CARTESIAN_POINT ( 'NONE',  ( 3.752267015613588906E-15, -4.381197846482986158, 2.812499999999997335 ) ) ;
#18317=CARTESIAN_POINT ( 'NONE',  ( 2.000000000000003997, -5.535898384862238508, 3.618749998770966148 ) ) ;
#18329=CARTESIAN_POINT ( 'NONE',  ( 3.735045420075836212E-15, -4.662447845253954171, 3.515624999385486227 ) ) ;
#18337=CIRCLE ( 'NONE', #11645, 4.000000000000000000 ) ;
#18338=CARTESIAN_POINT ( 'NONE',  ( -3.756430356249997882, -11.16877607737301226, 1.303124999385484095 ) ) ;
#18339=CARTESIAN_POINT ( 'NONE',  ( -3.999999999999997335, -11.30940107675849404, 3.412499999999996980 ) ) ;
#18342=CARTESIAN_POINT ( 'NONE',  ( -3.756430356249996105, -6.831223922626973533, 2.690624999385480276 ) ) ;
#18362=DIRECTION ( 'NONE',  ( -0.000000000000000000, -0.000000000000000000, -1.000000000000000000 ) ) ;
#18383=AXIS2_PLACEMENT_3D ( 'NONE', #22786, #4862, #3038 ) ;
#18393=AXIS2_PLACEMENT_3D ( 'NONE', #2267, #21751, #22132 ) ;
#18434=CARTESIAN_POINT ( 'NONE',  ( -3.756430356249996994, -8.999999999999992895, 3.178124999385484983 ) ) ;
#18473=CARTESIAN_POINT ( 'NONE',  ( 3.756430356250003655, -8.999999999999992895, 2.053124999385484095 ) ) ;
#18479=CARTESIAN_POINT ( 'NONE',  ( 3.735045420075836212E-15, -4.662447845253954171, 2.053124999385483207 ) ) ;
#18485=CARTESIAN_POINT ( 'NONE',  ( -3.756430356249997438, -11.16877607737301048, 1.415624999385483029 ) ) ;
#18570=CARTESIAN_POINT ( 'NONE',  ( -3.756430356249997882, -11.16877607737301226, 1.865624999385482985 ) ) ;
#18595=CARTESIAN_POINT ( 'NONE',  ( -3.756430356249996994, -8.999999999999992895, 3.178124999385484983 ) ) ;
#18600=CARTESIAN_POINT ( 'NONE',  ( 3.752267015613588906E-15, -4.381197846482986158, 0.5624999999999986677 ) ) ;
#18602=CARTESIAN_POINT ( 'NONE',  ( -1.878215178124998497, -12.25316411605951927, 1.340624999385482630 ) ) ;
#18604=CARTESIAN_POINT ( 'NONE',  ( -1.999999999999998224, -12.46410161513774639, 3.449999999999998401 ) ) ;
#18608=CARTESIAN_POINT ( 'NONE',  ( 3.756430356250003211, -6.831223922626973533, 1.640624999385484895 ) ) ;
#18617=VERTEX_POINT ( 'NONE', #21432 ) ;
#18622=( BOUNDED_CURVE ( )  B_SPLINE_CURVE ( 2, ( #17134, #23394, #11610, #11224, #15294, #7571, #23262 ),
 .UNSPECIFIED., .F., .F. ) 
 B_SPLINE_CURVE_WITH_KNOTS ( ( 3, 2, 2, 3 ),
 ( 0.9500000000000003997, 0.9666666666666670071, 0.9833333333333333925, 1.000000000000000000 ),
 .UNSPECIFIED. ) 
 CURVE ( )  GEOMETRIC_REPRESENTATION_ITEM ( )  RATIONAL_B_SPLINE_CURVE ( ( 0.9999999999999964473, 0.8660254037844422603, 1.000000000000000000, 0.8660254037844387076, 1.000000000000000000, 0.8660254037844387076, 1.000000000000000000 ) ) 
 REPRESENTATION_ITEM ( '' )  );
#18654=ADVANCED_FACE ( 'NONE', ( #23643 ), #5854, .T. ) ;
#18667=ORIENTED_EDGE ( 'NONE', *, *, #9765, .F. ) ;
#18682=CARTESIAN_POINT ( 'NONE',  ( -3.756430356249996994, -8.999999999999992895, 2.728124999385482585 ) ) ;
#18686=CARTESIAN_POINT ( 'NONE',  ( 4.000000000000003553, -8.999999999999992895, 0.8437499987709664584 ) ) ;
#18693=DIRECTION ( 'NONE',  ( 0.000000000000000000, 0.000000000000000000, 1.000000000000000000 ) ) ;
#18697=EDGE_CURVE ( 'NONE', #3646, #1770, #14115, .T. ) ;
#18704=EDGE_LOOP ( 'NONE', ( #16067, #10120 ) ) ;
#18710=CARTESIAN_POINT ( 'NONE',  ( 2.672651547586948120E-15, -13.33755215474602984, 1.378124999385482274 ) ) ;
#18716=CARTESIAN_POINT ( 'NONE',  ( 3.756430356250004099, -6.831223922626973533, 3.778124999385480631 ) ) ;
#18722=CARTESIAN_POINT ( 'NONE',  ( 3.756430356250003211, -6.831223922626973533, 2.990624999385483651 ) ) ;
#18780=CARTESIAN_POINT ( 'NONE',  ( -1.878215178124998497, -12.25316411605951927, 4.040624999385483918 ) ) ;
#18797=CARTESIAN_POINT ( 'NONE',  ( 2.000000000000000888, -12.46410161513774817, 3.075000000000001510 ) ) ;
#18818=CARTESIAN_POINT ( 'NONE',  ( 2.672651547586948120E-15, -13.33755215474602984, 1.490624999385481209 ) ) ;
#18846=AXIS2_PLACEMENT_3D ( 'NONE', #5178, #13154, #3197 ) ;
#18847=EDGE_CURVE ( 'NONE', #22527, #12823, #16108, .T. ) ;
#18854=CARTESIAN_POINT ( 'NONE',  ( -1.878215178124995832, -5.746835883940462963, 4.453124999385483562 ) ) ;
#18855=CARTESIAN_POINT ( 'NONE',  ( -3.999999999999996003, -6.690598923241487306, 0.5812499987709676130 ) ) ;
#18860=VECTOR ( 'NONE', #8271, 999.9999999999998863 ) ;
#18863=CARTESIAN_POINT ( 'NONE',  ( -1.878215178124998497, -12.25316411605951927, 3.140624999385482230 ) ) ;
#18864=CYLINDRICAL_SURFACE ( 'NONE', #18383, 4.000000000000000000 ) ;
#18865=CARTESIAN_POINT ( 'NONE',  ( -3.999999999999997335, -11.30940107675849404, 4.312500000000000000 ) ) ;
#18868=CARTESIAN_POINT ( 'NONE',  ( 2.672651547586948120E-15, -13.33755215474603162, 2.840624999385484628 ) ) ;
#18880=AXIS2_PLACEMENT_3D ( 'NONE', #5199, #5447, #3490 ) ;
#18890=CYLINDRICAL_SURFACE ( 'NONE', #9626, 4.000000000000000000 ) ;
#18891=EDGE_CURVE ( 'NONE', #23645, #9327, #17783, .T. ) ;
#18928=EDGE_CURVE ( 'NONE', #523, #20603, #3417, .T. ) ;
#18929=DIRECTION ( 'NONE',  ( -0.000000000000000000, -0.000000000000000000, -1.000000000000000000 ) ) ;
#18949=CARTESIAN_POINT ( 'NONE',  ( -1.878215178124995832, -5.746835883940462963, 4.453124999385483562 ) ) ;
#18958=ADVANCED_FACE ( 'NONE', ( #2937 ), #19621, .T. ) ;
#18980=CARTESIAN_POINT ( 'NONE',  ( 2.672651547586948120E-15, -13.33755215474602984, 4.190624999385483385 ) ) ;
#18985=CARTESIAN_POINT ( 'NONE',  ( -3.756430356249995661, -6.831223922626973533, 4.378124999385480720 ) ) ;
#18986=CARTESIAN_POINT ( 'NONE',  ( 4.000000000000003553, -8.999999999999992895, 4.500000000000000888 ) ) ;
#18991=CARTESIAN_POINT ( 'NONE',  ( -3.756430356249996105, -6.831223922626973533, 4.040624999385483918 ) ) ;
#19020=EDGE_CURVE ( 'NONE', #2372, #20735, #13622, .T. ) ;
#19023=CARTESIAN_POINT ( 'NONE',  ( 3.735045420075836212E-15, -4.662447845253954171, 0.2531249993854848279 ) ) ;
#19065=CARTESIAN_POINT ( 'NONE',  ( 2.672651547586948120E-15, -13.33755215474603162, 0.4781249993854826963 ) ) ;
#19067=CARTESIAN_POINT ( 'NONE',  ( 3.756430356250004099, -6.831223922626973533, 3.890624999385483562 ) ) ;
#19096=EDGE_CURVE ( 'NONE', #2372, #20798, #9755, .T. ) ;
#19097=CARTESIAN_POINT ( 'NONE',  ( -3.756430356249995661, -6.831223922626973533, 4.040624999385483918 ) ) ;
#19098=CARTESIAN_POINT ( 'NONE',  ( -3.999999999999996003, -6.690598923241487306, 1.931249998770966814 ) ) ;
#19103=CARTESIAN_POINT ( 'NONE',  ( 2.672651547586948120E-15, -13.33755215474602984, 4.078124999385480010 ) ) ;
#19105=CARTESIAN_POINT ( 'NONE',  ( 3.756430356250003655, -8.999999999999992895, 4.753124999385485161 ) ) ;
#19108=CARTESIAN_POINT ( 'NONE',  ( 4.000000000000003553, -8.999999999999992895, 0.3937499987709675020 ) ) ;
#19157=VECTOR ( 'NONE', #7666, 1000.000000000000000 ) ;
#19181=VERTEX_POINT ( 'NONE', #20003 ) ;
#19186=CARTESIAN_POINT ( 'NONE',  ( 2.672651547586948120E-15, -13.33755215474603162, 1.828124999385482008 ) ) ;
#19223=CARTESIAN_POINT ( 'NONE',  ( 1.878215178125000939, -12.25316411605952283, 1.415624999385481253 ) ) ;
#19224=CARTESIAN_POINT ( 'NONE',  ( -3.999999999999997335, -11.30940107675849404, 1.106249998770969301 ) ) ;
#19227=CARTESIAN_POINT ( 'NONE',  ( -1.999999999999998224, -12.46410161513774639, 3.843749998770965792 ) ) ;
#19230=CARTESIAN_POINT ( 'NONE',  ( -3.756430356249996994, -8.999999999999992895, 3.065624999385483385 ) ) ;
#19241=CARTESIAN_POINT ( 'NONE',  ( 4.000000000000018652, -6.690598923241496188, 4.031249998770966236 ) ) ;
#19258=VECTOR ( 'NONE', #16849, 1000.000000000000000 ) ;
#19273=EDGE_CURVE ( 'NONE', #18617, #11292, #18337, .T. ) ;
#19306=CARTESIAN_POINT ( 'NONE',  ( -3.999999999999996447, -8.999999999999992895, 2.868749998770965703 ) ) ;
#19310=CARTESIAN_POINT ( 'NONE',  ( 4.000000000000003553, -8.999999999999992895, 3.149999999999999911 ) ) ;
#19328=CARTESIAN_POINT ( 'NONE',  ( 3.735045420075836212E-15, -4.662447845253954171, 1.603124999385479921 ) ) ;
#19343=DIRECTION ( 'NONE',  ( -0.000000000000000000, -0.000000000000000000, 1.000000000000000000 ) ) ;
#19358=CARTESIAN_POINT ( 'NONE',  ( -1.878215178124995832, -5.746835883940462963, 2.540624999385482141 ) ) ;
#19359=CARTESIAN_POINT ( 'NONE',  ( -3.999999999999996447, -8.999999999999992895, 1.068749998770966103 ) ) ;
#19365=CARTESIAN_POINT ( 'NONE',  ( 2.000000000000000888, -12.46410161513774817, 1.274999999999998357 ) ) ;
#19370=CARTESIAN_POINT ( 'NONE',  ( -3.756430356249996994, -8.999999999999992895, 4.078124999385482674 ) ) ;
#19372=CARTESIAN_POINT ( 'NONE',  ( 2.620986760973688460E-15, -13.61880215351699874, 4.781249998770964460 ) ) ;
#19393=DIRECTION ( 'NONE',  ( -0.000000000000000000, -0.000000000000000000, -1.000000000000000000 ) ) ;
#19418=EDGE_CURVE ( 'NONE', #14884, #13396, #18622, .T. ) ;
#19424=AXIS2_PLACEMENT_3D ( 'NONE', #12433, #16383, #6430 ) ;
#19431=EDGE_CURVE ( 'NONE', #16617, #19775, #11363, .T. ) ;
#19447=CARTESIAN_POINT ( 'NONE',  ( 1.878215178125000939, -12.25316411605952283, 1.415624999385481253 ) ) ;
#19451=CARTESIAN_POINT ( 'NONE',  ( -3.756430356249996994, -8.999999999999992895, 3.628124999385483829 ) ) ;
#19478=CARTESIAN_POINT ( 'NONE',  ( -3.756430356249995661, -6.831223922626973533, 3.028124999385485072 ) ) ;
#19479=CARTESIAN_POINT ( 'NONE',  ( -3.999999999999997335, -11.30940107675849404, 2.906249998770968457 ) ) ;
#19482=DIRECTION ( 'NONE',  ( -0.000000000000000000, -0.000000000000000000, -1.000000000000000000 ) ) ;
#19483=CARTESIAN_POINT ( 'NONE',  ( 2.000000000000003997, -5.535898384862238508, 1.424999999999999156 ) ) ;
#19486=CARTESIAN_POINT ( 'NONE',  ( -3.999999999999996447, -8.999999999999992895, 18.00000000000000000 ) ) ;
#19491=DIRECTION ( 'NONE',  ( -1.000000000000000000, 0.000000000000000000, 0.000000000000000000 ) ) ;
#19495=EDGE_LOOP ( 'NONE', ( #6428, #11201, #20388, #23032 ) ) ;
#19505=CARTESIAN_POINT ( 'NONE',  ( -1.878215178124995832, -5.746835883940462963, 1.303124999385483429 ) ) ;
#19511=EDGE_CURVE ( 'NONE', #6676, #12074, #21176, .T. ) ;
#19524=EDGE_LOOP ( 'NONE', ( #934, #2500 ) ) ;
#19562=EDGE_LOOP ( 'NONE', ( #3116, #17620, #22645, #14020, #2490 ) ) ;
#19567=CARTESIAN_POINT ( 'NONE',  ( -1.878215178124998497, -12.25316411605951927, 0.8906249993854836733 ) ) ;
#19599=( BOUNDED_CURVE ( )  B_SPLINE_CURVE ( 2, ( #17677, #23674, #5751, #13738, #21715, #3799, #11 ),
 .UNSPECIFIED., .F., .F. ) 
 B_SPLINE_CURVE_WITH_KNOTS ( ( 3, 2, 2, 3 ),
 ( 0.4499999999999998446, 0.4666666666666665075, 0.4833333333333331150, 0.4999999999999997780 ),
 .UNSPECIFIED. ) 
 CURVE ( )  GEOMETRIC_REPRESENTATION_ITEM ( )  RATIONAL_B_SPLINE_CURVE ( ( 1.000000000000001332, 0.8660254037844373753, 1.000000000000000000, 0.8660254037844387076, 1.000000000000000000, 0.8660254037844404840, 0.9999999999999982236 ) ) 
 REPRESENTATION_ITEM ( '' )  );
#19607=CARTESIAN_POINT ( 'NONE',  ( -1.878215178124998497, -12.25316411605951927, 2.240624999385484095 ) ) ;
#19608=CARTESIAN_POINT ( 'NONE',  ( 4.000000000000001776, -11.30940107675849760, 1.706249998770968945 ) ) ;
#19613=CARTESIAN_POINT ( 'NONE',  ( -3.999999999999997335, -11.30940107675849404, 2.962499999999996803 ) ) ;
#19621=CYLINDRICAL_SURFACE ( 'NONE', #792, 4.000000000000000000 ) ;
#19662=ORIENTED_EDGE ( 'NONE', *, *, #3860, .F. ) ;
#19708=CARTESIAN_POINT ( 'NONE',  ( 1.878215178125004048, -5.746835883940462963, 3.365624999385481875 ) ) ;
#19711=( LENGTH_UNIT ( ) NAMED_UNIT ( * ) SI_UNIT ( .MILLI., .METRE. ) );
#19746=CARTESIAN_POINT ( 'NONE',  ( -3.756430356249997882, -11.16877607737301226, 3.103124999385483029 ) ) ;
#19747=CARTESIAN_POINT ( 'NONE',  ( 2.000000000000000888, -12.46410161513774817, 4.368749998770966592 ) ) ;
#19749=EDGE_CURVE ( 'NONE', #24155, #25772, #2174, .T. ) ;
#19754=CARTESIAN_POINT ( 'NONE',  ( 2.000000000000003997, -5.535898384862238508, 1.875000000000001776 ) ) ;
#19769=DIRECTION ( 'NONE',  ( 0.000000000000000000, 0.000000000000000000, 1.000000000000000000 ) ) ;
#19770=EDGE_LOOP ( 'NONE', ( #16854, #2458, #17964, #11796 ) ) ;
#19775=VERTEX_POINT ( 'NONE', #21525 ) ;
#19814=DIRECTION ( 'NONE',  ( -0.000000000000000000, -0.000000000000000000, -1.000000000000000000 ) ) ;
#19828=CARTESIAN_POINT ( 'NONE',  ( 1.878215178125004048, -5.746835883940462963, 4.265624999385483562 ) ) ;
#19829=SHAPE_REPRESENTATION ( 'stem', ( #21036 ), #5183 ) ;
#19831=EDGE_CURVE ( 'NONE', #9030, #6676, #5252, .T. ) ;
#19832=CARTESIAN_POINT ( 'NONE',  ( 2.000000000000000888, -12.46410161513774817, 3.974999999999999201 ) ) ;
#19862=CARTESIAN_POINT ( 'NONE',  ( 1.878215178125004048, -5.746835883940462963, 2.915624999385482585 ) ) ;
#19863=CARTESIAN_POINT ( 'NONE',  ( -1.999999999999995781, -5.535898384862237620, 4.143749998770966947 ) ) ;
#19866=CARTESIAN_POINT ( 'NONE',  ( -1.999999999999998224, -12.46410161513774639, 0.7500000000000006661 ) ) ;
#19867=CARTESIAN_POINT ( 'NONE',  ( -1.999999999999998224, -12.46410161513774639, 2.999999999999999112 ) ) ;
#19891=CARTESIAN_POINT ( 'NONE',  ( 2.672651547586948120E-15, -13.33755215474602984, 1.040624999385485472 ) ) ;
#19892=CARTESIAN_POINT ( 'NONE',  ( 4.000000000000003553, -8.999999999999992895, 1.293749998770969079 ) ) ;
#19898=CARTESIAN_POINT ( 'NONE',  ( 1.878215178125004048, -5.746835883940462963, 0.7781249993854856273 ) ) ;
#19912=EDGE_CURVE ( 'NONE', #16478, #2372, #16801, .T. ) ;
#19949=CARTESIAN_POINT ( 'NONE',  ( 1.878215178125004048, -5.746835883940462963, 3.815624999385484273 ) ) ;
#19987=CARTESIAN_POINT ( 'NONE',  ( -3.999999999999997335, -11.30940107675849404, 4.256249998770964105 ) ) ;
#20003=CARTESIAN_POINT ( 'NONE',  ( 4.000000000000003553, -8.999999999999992895, 1.743749998770967924 ) ) ;
#20006=CARTESIAN_POINT ( 'NONE',  ( -3.999999999999996447, -8.999999999999992895, 1.574999999999999956 ) ) ;
#20026=DIRECTION ( 'NONE',  ( -1.000000000000000000, 0.000000000000000000, 0.000000000000000000 ) ) ;
#20028=CIRCLE ( 'NONE', #834, 4.000000000000000000 ) ;
#20029=CARTESIAN_POINT ( 'NONE',  ( -3.756430356249995661, -6.831223922626973533, 0.7781249993854825187 ) ) ;
#20060=CARTESIAN_POINT ( 'NONE',  ( 2.620986760973688460E-15, -13.61880215351699874, 1.181249998770967258 ) ) ;
#20087=CARTESIAN_POINT ( 'NONE',  ( -1.878215178124995832, -5.746835883940462963, 2.540624999385482141 ) ) ;
#20090=SURFACE_STYLE_USAGE ( .BOTH. , #4139 ) ;
#20108=CARTESIAN_POINT ( 'NONE',  ( 4.000000000000003553, -8.999999999999992895, 1.350000000000000533 ) ) ;
#20126=CARTESIAN_POINT ( 'NONE',  ( -3.999999999999997335, -11.30940107675849404, 3.356249998770967746 ) ) ;
#20146=ORIENTED_EDGE ( 'NONE', *, *, #19020, .F. ) ;
#20158=CARTESIAN_POINT ( 'NONE',  ( 1.878215178125004048, -5.746835883940462963, 3.028124999385484184 ) ) ;
#20163=CARTESIAN_POINT ( 'NONE',  ( 1.878215178125004048, -5.746835883940462963, 2.465624999385483740 ) ) ;
#20167=CARTESIAN_POINT ( 'NONE',  ( 2.000000000000000888, -12.46410161513774817, 3.525000000000000355 ) ) ;
#20216=CARTESIAN_POINT ( 'NONE',  ( 3.756430356250002323, -11.16877607737301403, 3.253124999385482941 ) ) ;
#20225=DIRECTION ( 'NONE',  ( -0.000000000000000000, -0.000000000000000000, -1.000000000000000000 ) ) ;
#20228=ORIENTED_EDGE ( 'NONE', *, *, #9005, .F. ) ;
#20250=CARTESIAN_POINT ( 'NONE',  ( 1.878215178125000939, -12.25316411605952283, 4.565624999385481608 ) ) ;
#20251=CARTESIAN_POINT ( 'NONE',  ( 3.756430356250002323, -11.16877607737301226, 0.6656249993854835845 ) ) ;
#20264=CARTESIAN_POINT ( 'NONE',  ( 2.620986760973688460E-15, -13.61880215351699874, 1.687500000000000000 ) ) ;
#20282=CARTESIAN_POINT ( 'NONE',  ( -1.878215178124998497, -12.25316411605951927, 3.253124999385483829 ) ) ;
#20289=CARTESIAN_POINT ( 'NONE',  ( -1.878215178124995832, -5.746835883940462963, 2.090624999385483296 ) ) ;
#20293=CARTESIAN_POINT ( 'NONE',  ( 1.878215178125000939, -12.25316411605952283, 2.428124999385484539 ) ) ;
#20301=ORIENTED_EDGE ( 'NONE', *, *, #22382, .T. ) ;
#20318=ADVANCED_FACE ( 'NONE', ( #10623, #22276 ), #16263, .F. ) ;
#20345=FACE_OUTER_BOUND ( 'NONE', #13371, .T. ) ;
#20372=CARTESIAN_POINT ( 'NONE',  ( -1.878215178124995832, -5.746835883940462963, 1.753124999385485827 ) ) ;
#20374=CARTESIAN_POINT ( 'NONE',  ( 3.752267015613588906E-15, -4.381197846482986158, 1.856249998770964638 ) ) ;
#20375=CARTESIAN_POINT ( 'NONE',  ( -1.999999999999995781, -5.535898384862237620, 3.750000000000000000 ) ) ;
#20388=ORIENTED_EDGE ( 'NONE', *, *, #9765, .T. ) ;
#20389=CARTESIAN_POINT ( 'NONE',  ( 4.000000000000003553, -8.999999999999992895, 18.00000000000000000 ) ) ;
#20403=CARTESIAN_POINT ( 'NONE',  ( 2.672651547586948120E-15, -13.33755215474602984, 1.940624999385484717 ) ) ;
#20405=CARTESIAN_POINT ( 'NONE',  ( 4.000000000000003553, -6.690598923241489970, 0.4312499987709677018 ) ) ;
#20409=VECTOR ( 'NONE', #10039, 1000.000000000000000 ) ;
#20410=CARTESIAN_POINT ( 'NONE',  ( -3.756430356249997882, -11.16877607737301226, 0.8531249993854844726 ) ) ;
#20411=CARTESIAN_POINT ( 'NONE',  ( -1.999999999999998224, -12.46410161513774639, 4.349999999999999645 ) ) ;
#20415=CARTESIAN_POINT ( 'NONE',  ( -1.878215178124995832, -5.746835883940462963, 0.8531249993854843616 ) ) ;
#20423=ORIENTED_EDGE ( 'NONE', *, *, #7955, .F. ) ;
#20435=( BOUNDED_CURVE ( )  B_SPLINE_CURVE ( 2, ( #22583, #22718, #4519, #353, #12774, #6367, #737 ),
 .UNSPECIFIED., .F., .F. ) 
 B_SPLINE_CURVE_WITH_KNOTS ( ( 3, 2, 2, 3 ),
 ( 0.2000000000000003719, 0.2166666666666670071, 0.2333333333333336423, 0.2500000000000002776 ),
 .UNSPECIFIED. ) 
 CURVE ( )  GEOMETRIC_REPRESENTATION_ITEM ( )  RATIONAL_B_SPLINE_CURVE ( ( 0.9999999999999971134, 0.8660254037844415942, 1.000000000000000000, 0.8660254037844387076, 1.000000000000000000, 0.8660254037844364872, 1.000000000000002220 ) ) 
 REPRESENTATION_ITEM ( '' )  );
#20467=ORIENTED_EDGE ( 'NONE', *, *, #10589, .T. ) ;
#20494=CARTESIAN_POINT ( 'NONE',  ( -3.999999999999959144, -11.30940107675851891, 1.162499999999999423 ) ) ;
#20514=EDGE_CURVE ( 'NONE', #20798, #19181, #24760, .T. ) ;
#20516=CARTESIAN_POINT ( 'NONE',  ( -1.878215178124998497, -12.25316411605951927, 1.453124999385484228 ) ) ;
#20531=CARTESIAN_POINT ( 'NONE',  ( -4.000000000000026645, -6.690598923241505958, 2.887499999999999734 ) ) ;
#20552=CARTESIAN_POINT ( 'NONE',  ( -3.756430356249997882, -11.16877607737301226, 2.315624999385482496 ) ) ;
#20559=CARTESIAN_POINT ( 'NONE',  ( 4.000000000000030198, -6.690598923241506846, 0.4874999999999962697 ) ) ;
#20560=CARTESIAN_POINT ( 'NONE',  ( 3.756430356250004099, -6.831223922626973533, 2.878124999385481608 ) ) ;
#20565=CARTESIAN_POINT ( 'NONE',  ( 3.756430356250003655, -8.999999999999992895, 2.503124999385482941 ) ) ;
#20584=STYLED_ITEM('',(#25907),#4802);
#20603=VERTEX_POINT ( 'NONE', #17176 ) ;
#20604=( BOUNDED_SURFACE ( )  B_SPLINE_SURFACE ( 1, 2, ( 
 ( #16770, #20405, #12966, #14806, #20947, #18855, #8533, #16514, #24476, #17289, #25504, #3269, #23546, #15441, #13222, #11244, #1711, #21192, #19359, #19224, #5499, #1573, #3153, #21328, #15578, #17152, #3537, #25638, #1324, #11119, #23414, #9304, #3406, #7211, #5126, #19608, #13492, #11631, #1182, #25254, #13352, #19098, #9162, #21076, #7333, #15313, #9684, #7454, #21460, #9544, #25123, #17530, #15063, #15193, #17405, #11384, #23163, #23038, #5243, #23281, #1454, #17670, #25370, #13102, #11508, #5363, #9425, #19479, #7593, #5629, #13610, #21575, #3654, #21967, #9808, #10185, #25756, #6136, #12152, #20126, #17790, #21842, #1961, #23668, #22085, #18183, #7838, #13994, #2228, #3923, #15822, #23932, #12010, #5883, #23794, #11894, #11769, #13867, #7978, #6014, #19863, #24052, #6267, #19987, #2092, #14259, #19747, #5745, #18058, #9925, #3, #7719, #266, #15702, #17912, #3792, #18299, #4043, #22226, #10058, #15964 ),
 ( #16089, #4311, #142, #8115, #14121, #13726, #16211, #4174, #8232, #24179, #12286, #20251, #2349, #10304, #21707, #1846, #8887, #770, #24444, #22477, #12929, #6521, #4706, #14505, #16732, #4948, #652, #10571, #20776, #10964, #8500, #22347, #20516, #18818, #4556, #22868, #14894, #4432, #12539, #12405, #20372, #908, #6788, #18570, #6649, #8620, #2612, #16599, #12802, #10695, #24703, #392, #16870, #24560, #16482, #14391, #14637, #22617, #20908, #12679, #2995, #2467, #8361, #2855, #20650, #2732, #18682, #8742, #10824, #14773, #24836, #10440, #6911, #22748, #4825, #16350, #24319, #6399, #18434, #528, #21542, #5214, #5463, #7177, #15023, #9510, #7554, #11209, #23379, #25225, #19451, #3506, #17492, #21425, #25467, #13068, #7305, #19067, #15544, #1542, #1034, #17376, #5332, #3371, #13457, #25091, #5598, #15165, #7036, #25341, #17116, #23512, #18949, #3625, #15281, #7420, #21046, #11476, #23002, #13577, #23247 ) ),
 .UNSPECIFIED., .F., .F., .T. ) 
 B_SPLINE_SURFACE_WITH_KNOTS ( ( 2, 2 ),
 ( 3, 2, 2, 2, 2, 2, 2, 2, 2, 2, 2, 2, 2, 2, 2, 2, 2, 2, 2, 2, 2, 2, 2, 2, 2, 2, 2, 2, 2, 2, 2, 2, 2, 2, 2, 2, 2, 2, 2, 2, 2, 2, 2, 2, 2, 2, 2, 2, 2, 2, 2, 2, 2, 2, 2, 2, 2, 2, 2, 2, 3 ),
 ( 0.000000000000000000, 1.000000000000000000 ),
 ( 0.000000000000000000, 0.01666666666666666644, 0.03333333333333333287, 0.05000000000000000278, 0.06666666666666666574, 0.08333333333333332871, 0.1000000000000000056, 0.1166666666666666685, 0.1333333333333333315, 0.1499999999999999944, 0.1666666666666666574, 0.1833333333333333204, 0.2000000000000000111, 0.2166666666666666741, 0.2333333333333333370, 0.2500000000000000000, 0.2666666666666666630, 0.2833333333333333259, 0.2999999999999999889, 0.3166666666666666519, 0.3333333333333333148, 0.3499999999999999778, 0.3666666666666666408, 0.3833333333333333592, 0.4000000000000000222, 0.4166666666666666852, 0.4333333333333333481, 0.4500000000000000111, 0.4666666666666666741, 0.4833333333333333370, 0.5000000000000000000, 0.5166666666666667185, 0.5333333333333333259, 0.5500000000000000444, 0.5666666666666666519, 0.5833333333333333703, 0.5999999999999999778, 0.6166666666666666963, 0.6333333333333333037, 0.6500000000000000222, 0.6666666666666666297, 0.6833333333333333481, 0.6999999999999999556, 0.7166666666666666741, 0.7333333333333332815, 0.7500000000000000000, 0.7666666666666667185, 0.7833333333333333259, 0.8000000000000000444, 0.8166666666666666519, 0.8333333333333333703, 0.8499999999999999778, 0.8666666666666666963, 0.8833333333333333037, 0.9000000000000000222, 0.9166666666666666297, 0.9333333333333333481, 0.9499999999999999556, 0.9666666666666666741, 0.9833333333333332815, 1.000000000000000000 ),
 .UNSPECIFIED. ) 
 GEOMETRIC_REPRESENTATION_ITEM ( )  RATIONAL_B_SPLINE_SURFACE ( (
 ( 1.000000000000000000, 0.8660254037844387076, 1.000000000000000000, 0.8660254037844387076, 1.000000000000000000, 0.8660254037844387076, 1.000000000000000000, 0.8660254037844387076, 1.000000000000000000, 0.8660254037844387076, 1.000000000000000000, 0.8660254037844387076, 1.000000000000000000, 0.8660254037844387076, 1.000000000000000000, 0.8660254037844387076, 1.000000000000000000, 0.8660254037844387076, 1.000000000000000000, 0.8660254037844387076, 1.000000000000000000, 0.8660254037844387076, 1.000000000000000000, 0.8660254037844387076, 1.000000000000000000, 0.8660254037844387076, 1.000000000000000000, 0.8660254037844387076, 1.000000000000000000, 0.8660254037844387076, 1.000000000000000000, 0.8660254037844387076, 1.000000000000000000, 0.8660254037844387076, 1.000000000000000000, 0.8660254037844387076, 1.000000000000000000, 0.8660254037844387076, 1.000000000000000000, 0.8660254037844387076, 1.000000000000000000, 0.8660254037844387076, 1.000000000000000000, 0.8660254037844387076, 1.000000000000000000, 0.8660254037844387076, 1.000000000000000000, 0.8660254037844387076, 1.000000000000000000, 0.8660254037844387076, 1.000000000000000000, 0.8660254037844387076, 1.000000000000000000, 0.8660254037844387076, 1.000000000000000000, 0.8660254037844387076, 1.000000000000000000, 0.8660254037844387076, 1.000000000000000000, 0.8660254037844387076, 1.000000000000000000, 0.8660254037844387076, 1.000000000000000000, 0.8660254037844387076, 1.000000000000000000, 0.8660254037844387076, 1.000000000000000000, 0.8660254037844387076, 1.000000000000000000, 0.8660254037844387076, 1.000000000000000000, 0.8660254037844387076, 1.000000000000000000, 0.8660254037844387076, 1.000000000000000000, 0.8660254037844387076, 1.000000000000000000, 0.8660254037844387076, 1.000000000000000000, 0.8660254037844387076, 1.000000000000000000, 0.8660254037844387076, 1.000000000000000000, 0.8660254037844387076, 1.000000000000000000, 0.8660254037844387076, 1.000000000000000000, 0.8660254037844387076, 1.000000000000000000, 0.8660254037844387076, 1.000000000000000000, 0.8660254037844387076, 1.000000000000000000, 0.8660254037844387076, 1.000000000000000000, 0.8660254037844387076, 1.000000000000000000, 0.8660254037844387076, 1.000000000000000000, 0.8660254037844387076, 1.000000000000000000, 0.8660254037844387076, 1.000000000000000000, 0.8660254037844387076, 1.000000000000000000, 0.8660254037844387076, 1.000000000000000000, 0.8660254037844387076, 1.000000000000000000, 0.8660254037844387076, 1.000000000000000000, 0.8660254037844387076, 1.000000000000000000, 0.8660254037844387076, 1.000000000000000000, 0.8660254037844387076, 1.000000000000000000, 0.8660254037844387076, 1.000000000000000000, 0.8660254037844387076, 1.000000000000000000),
 ( 1.000000000000000000, 0.8660254037844387076, 1.000000000000000000, 0.8660254037844387076, 1.000000000000000000, 0.8660254037844387076, 1.000000000000000000, 0.8660254037844387076, 1.000000000000000000, 0.8660254037844387076, 1.000000000000000000, 0.8660254037844387076, 1.000000000000000000, 0.8660254037844387076, 1.000000000000000000, 0.8660254037844387076, 1.000000000000000000, 0.8660254037844387076, 1.000000000000000000, 0.8660254037844387076, 1.000000000000000000, 0.8660254037844387076, 1.000000000000000000, 0.8660254037844387076, 1.000000000000000000, 0.8660254037844387076, 1.000000000000000000, 0.8660254037844387076, 1.000000000000000000, 0.8660254037844387076, 1.000000000000000000, 0.8660254037844387076, 1.000000000000000000, 0.8660254037844387076, 1.000000000000000000, 0.8660254037844387076, 1.000000000000000000, 0.8660254037844387076, 1.000000000000000000, 0.8660254037844387076, 1.000000000000000000, 0.8660254037844387076, 1.000000000000000000, 0.8660254037844387076, 1.000000000000000000, 0.8660254037844387076, 1.000000000000000000, 0.8660254037844387076, 1.000000000000000000, 0.8660254037844387076, 1.000000000000000000, 0.8660254037844387076, 1.000000000000000000, 0.8660254037844387076, 1.000000000000000000, 0.8660254037844387076, 1.000000000000000000, 0.8660254037844387076, 1.000000000000000000, 0.8660254037844387076, 1.000000000000000000, 0.8660254037844387076, 1.000000000000000000, 0.8660254037844387076, 1.000000000000000000, 0.8660254037844387076, 1.000000000000000000, 0.8660254037844387076, 1.000000000000000000, 0.8660254037844387076, 1.000000000000000000, 0.8660254037844387076, 1.000000000000000000, 0.8660254037844387076, 1.000000000000000000, 0.8660254037844387076, 1.000000000000000000, 0.8660254037844387076, 1.000000000000000000, 0.8660254037844387076, 1.000000000000000000, 0.8660254037844387076, 1.000000000000000000, 0.8660254037844387076, 1.000000000000000000, 0.8660254037844387076, 1.000000000000000000, 0.8660254037844387076, 1.000000000000000000, 0.8660254037844387076, 1.000000000000000000, 0.8660254037844387076, 1.000000000000000000, 0.8660254037844387076, 1.000000000000000000, 0.8660254037844387076, 1.000000000000000000, 0.8660254037844387076, 1.000000000000000000, 0.8660254037844387076, 1.000000000000000000, 0.8660254037844387076, 1.000000000000000000, 0.8660254037844387076, 1.000000000000000000, 0.8660254037844387076, 1.000000000000000000, 0.8660254037844387076, 1.000000000000000000, 0.8660254037844387076, 1.000000000000000000, 0.8660254037844387076, 1.000000000000000000, 0.8660254037844387076, 1.000000000000000000, 0.8660254037844387076, 1.000000000000000000, 0.8660254037844387076, 1.000000000000000000, 0.8660254037844387076, 1.000000000000000000) ) ) 
 REPRESENTATION_ITEM ( '' )  SURFACE ( )  );
#20626=CYLINDRICAL_SURFACE ( 'NONE', #4210, 4.000000000000000000 ) ;
#20632=CARTESIAN_POINT ( 'NONE',  ( -1.999999999999998224, -12.46410161513774639, 1.199999999999999734 ) ) ;
#20643=APPLICATION_CONTEXT ( 'automotive_design' ) ;
#20650=CARTESIAN_POINT ( 'NONE',  ( -1.878215178124995832, -5.746835883940462963, 2.653124999385483740 ) ) ;
#20654=CARTESIAN_POINT ( 'NONE',  ( 4.000000000000003553, -8.999999999999992895, 1.743749998770967924 ) ) ;
#20674=ORIENTED_EDGE ( 'NONE', *, *, #18146, .T. ) ;
#20680=CARTESIAN_POINT ( 'NONE',  ( 3.756430356250002323, -11.16877607737301226, 2.465624999385482852 ) ) ;
#20686=CARTESIAN_POINT ( 'NONE',  ( -1.878215178124998497, -12.25316411605951927, 4.040624999385483918 ) ) ;
#20692=CARTESIAN_POINT ( 'NONE',  ( -3.756430356249997438, -11.16877607737301048, 2.765624999385486227 ) ) ;
#20693=CYLINDRICAL_SURFACE ( 'NONE', #18295, 4.000000000000000000 ) ;
#20735=VERTEX_POINT ( 'NONE', #9948 ) ;
#20756=CARTESIAN_POINT ( 'NONE',  ( 3.000000000000003997, -8.999999999999992895, 0.000000000000000000 ) ) ;
#20767=EDGE_CURVE ( 'NONE', #21696, #16617, #24581, .T. ) ;
#20775=CARTESIAN_POINT ( 'NONE',  ( 2.000000000000003997, -5.535898384862238508, 1.875000000000001776 ) ) ;
#20776=CARTESIAN_POINT ( 'NONE',  ( -1.878215178124995832, -5.746835883940462963, 1.303124999385483429 ) ) ;
#20782=CARTESIAN_POINT ( 'NONE',  ( 3.756430356250003655, -8.999999999999992895, 4.696874999385483918 ) ) ;
#20798=VERTEX_POINT ( 'NONE', #8609 ) ;
#20806=CARTESIAN_POINT ( 'NONE',  ( -3.756430356249997882, -11.16877607737301226, 4.115624999385481431 ) ) ;
#20812=CARTESIAN_POINT ( 'NONE',  ( 2.000000000000000888, -12.46410161513774817, 0.3750000000000003331 ) ) ;
#20817=CARTESIAN_POINT ( 'NONE',  ( -3.756430356249997438, -11.16877607737301048, 1.865624999385482985 ) ) ;
#20820=ORIENTED_EDGE ( 'NONE', *, *, #13948, .F. ) ;
#20854=CARTESIAN_POINT ( 'NONE',  ( 1.878215178125000939, -12.25316411605952283, 0.5156249993854833402 ) ) ;
#20876=CARTESIAN_POINT ( 'NONE',  ( 4.000000000000003553, -8.999999999999992895, 3.093749998770968457 ) ) ;
#20908=CARTESIAN_POINT ( 'NONE',  ( 1.878215178125000939, -12.25316411605952283, 2.428124999385484539 ) ) ;
#20936=ORIENTED_EDGE ( 'NONE', *, *, #3860, .T. ) ;
#20945=VECTOR ( 'NONE', #4628, 1000.000000000000000 ) ;
#20946=CARTESIAN_POINT ( 'NONE',  ( 3.756430356250003655, -8.999999999999992895, 4.303124999385482319 ) ) ;
#20947=CARTESIAN_POINT ( 'NONE',  ( -1.999999999999995781, -5.535898384862237620, 0.5437499987709683014 ) ) ;
#20954=CARTESIAN_POINT ( 'NONE',  ( 2.672651547586948120E-15, -13.33755215474602984, 3.178124999385481431 ) ) ;
#20955=ADVANCED_FACE ( 'NONE', ( #24691 ), #2114, .T. ) ;
#20957=CARTESIAN_POINT ( 'NONE',  ( 4.000000000000003553, -8.999999999999992895, 4.049999999999998046 ) ) ;
#20960=CARTESIAN_POINT ( 'NONE',  ( 1.878215178125000939, -12.25316411605952283, 3.328124999385485783 ) ) ;
#20961=DIRECTION ( 'NONE',  ( 0.000000000000000000, 0.000000000000000000, 1.000000000000000000 ) ) ;
#20962=CARTESIAN_POINT ( 'NONE',  ( 3.752267015613588906E-15, -4.381197846482986158, 4.106249998770967302 ) ) ;
#21005=VERTEX_POINT ( 'NONE', #10651 ) ;
#21036=AXIS2_PLACEMENT_3D ( 'NONE', #13353, #15703, #13223 ) ;
#21045=CARTESIAN_POINT ( 'NONE',  ( 1.878215178125000939, -12.25316411605952283, 0.5156249993854833402 ) ) ;
#21046=CARTESIAN_POINT ( 'NONE',  ( -1.878215178124998497, -12.25316411605951927, 4.603124999385483918 ) ) ;
#21053=CARTESIAN_POINT ( 'NONE',  ( -1.999999999999998224, -12.46410161513774639, 0.6937499987709692117 ) ) ;
#21075=CARTESIAN_POINT ( 'NONE',  ( 1.878215178125000939, -12.25316411605952283, 4.228124999385483918 ) ) ;
#21076=CARTESIAN_POINT ( 'NONE',  ( -3.999999999999997335, -11.30940107675849404, 2.006249998770964993 ) ) ;
#21080=CARTESIAN_POINT ( 'NONE',  ( 1.878215178125000939, -12.25316411605952283, 4.565624999385481608 ) ) ;
#21085=CARTESIAN_POINT ( 'NONE',  ( 3.756430356250002323, -11.16877607737301403, 4.715624999385485516 ) ) ;
#21087=CARTESIAN_POINT ( 'NONE',  ( -1.999999999999995781, -5.535898384862237620, 4.143749998770966947 ) ) ;
#21104=DIRECTION ( 'NONE',  ( -1.000000000000000000, 0.000000000000000000, 0.000000000000000000 ) ) ;
#21125=AXIS2_PLACEMENT_3D ( 'NONE', #7066, #15309, #9158 ) ;
#21129=APPLICATION_CONTEXT ( 'automotive_design' ) ;
#21131=SHAPE_DEFINITION_REPRESENTATION ( #2342, #19829 ) ;
#21160=CARTESIAN_POINT ( 'NONE',  ( -3.756430356249997438, -11.16877607737301048, 1.753124999385480276 ) ) ;
#21176=LINE ( 'NONE', #3248, #20409 ) ;
#21185=ORIENTED_EDGE ( 'NONE', *, *, #3848, .T. ) ;
#21191=CARTESIAN_POINT ( 'NONE',  ( 3.756430356250002323, -11.16877607737301226, 1.453124999385484228 ) ) ;
#21192=CARTESIAN_POINT ( 'NONE',  ( -3.999999999999996003, -6.690598923241487306, 1.031249998770967347 ) ) ;
#21198=CARTESIAN_POINT ( 'NONE',  ( -3.999999999999996003, -6.690598923241487306, 0.6374999999999966249 ) ) ;
#21203=CARTESIAN_POINT ( 'NONE',  ( 3.735045420075836212E-15, -4.662447845253954171, 4.415624999385481253 ) ) ;
#21246=ORIENTED_EDGE ( 'NONE', *, *, #2992, .F. ) ;
#21274=ORIENTED_EDGE ( 'NONE', *, *, #12394, .F. ) ;
#21286=CARTESIAN_POINT ( 'NONE',  ( 3.756430356250003655, -8.999999999999992895, 1.040624999385484584 ) ) ;
#21287=( BOUNDED_CURVE ( )  B_SPLINE_CURVE ( 2, ( #24872, #20559, #6952, #18600, #11005, #687, #14931 ),
 .UNSPECIFIED., .F., .F. ) 
 B_SPLINE_CURVE_WITH_KNOTS ( ( 3, 2, 2, 3 ),
 ( 0.09999999999999981126, 0.1166666666666664326, 0.1333333333333330539, 0.1499999999999996891 ),
 .UNSPECIFIED. ) 
 CURVE ( )  GEOMETRIC_REPRESENTATION_ITEM ( )  RATIONAL_B_SPLINE_CURVE ( ( 1.000000000000001776, 0.8660254037844372643, 1.000000000000000000, 0.8660254037844387076, 1.000000000000000000, 0.8660254037844411501, 0.9999999999999975575 ) ) 
 REPRESENTATION_ITEM ( '' )  );
#21300=CARTESIAN_POINT ( 'NONE',  ( -4.000000000000010658, -11.30940107675848694, 0.6562499987709652371 ) ) ;
#21303=DIRECTION ( 'NONE',  ( -0.8660254037844397068, 0.000000000000000000, -0.4999999999999983347 ) ) ;
#21318=EDGE_LOOP ( 'NONE', ( #11195, #10522, #14204, #14174 ) ) ;
#21327=CARTESIAN_POINT ( 'NONE',  ( 1.878215178125004048, -5.746835883940462963, 0.2156249993854816860 ) ) ;
#21328=CARTESIAN_POINT ( 'NONE',  ( 4.000000000000001776, -11.30940107675849760, 1.256249998770964993 ) ) ;
#21332=CARTESIAN_POINT ( 'NONE',  ( 4.000000000000001776, -11.30940107675849760, 1.762499999999997957 ) ) ;
#21337=CARTESIAN_POINT ( 'NONE',  ( 1.878215178125004048, -5.746835883940462963, 3.478124999385483029 ) ) ;
#21340=CARTESIAN_POINT ( 'NONE',  ( 3.999999999999942268, -6.690598923241455331, 3.131249998770967213 ) ) ;
#21376=DIRECTION ( 'NONE',  ( -0.000000000000000000, -0.000000000000000000, -1.000000000000000000 ) ) ;
#21418=ORIENTED_EDGE ( 'NONE', *, *, #11447, .F. ) ;
#21425=CARTESIAN_POINT ( 'NONE',  ( 2.672651547586948120E-15, -13.33755215474602984, 3.740624999385483651 ) ) ;
#21432=CARTESIAN_POINT ( 'NONE',  ( 4.000000000000003553, -8.999999999999992895, 18.00000000000000000 ) ) ;
#21459=CARTESIAN_POINT ( 'NONE',  ( 1.878215178125000939, -12.25316411605952283, 3.665624999385483473 ) ) ;
#21460=CARTESIAN_POINT ( 'NONE',  ( 4.000000000000003553, -8.999999999999992895, 2.193749998770967213 ) ) ;
#21466=CARTESIAN_POINT ( 'NONE',  ( -1.999999999999995781, -5.535898384862237620, 2.399999999999999467 ) ) ;
#21489=CYLINDRICAL_SURFACE ( 'NONE', #25549, 4.000000000000000000 ) ;
#21494=EDGE_CURVE ( 'NONE', #16478, #7351, #16278, .T. ) ;
#21525=CARTESIAN_POINT ( 'NONE',  ( 3.000000000000003997, -8.999999999999992895, 18.00000000000000000 ) ) ;
#21533=CARTESIAN_POINT ( 'NONE',  ( 4.000000000000003553, -8.999999999999992895, 0.4499999999999990119 ) ) ;
#21541=CARTESIAN_POINT ( 'NONE',  ( -1.878215178124995832, -5.746835883940462963, 0.2906249993854838065 ) ) ;
#21542=CARTESIAN_POINT ( 'NONE',  ( -1.878215178124998497, -12.25316411605951927, 3.253124999385483829 ) ) ;
#21574=CARTESIAN_POINT ( 'NONE',  ( -3.756430356249995661, -6.831223922626973533, 2.128124999385482052 ) ) ;
#21575=CARTESIAN_POINT ( 'NONE',  ( 4.000000000000001776, -11.30940107675849760, 3.056249998770964371 ) ) ;
#21580=CARTESIAN_POINT ( 'NONE',  ( 3.752267015613588906E-15, -4.381197846482986158, 1.012499999999998401 ) ) ;
#21589=CARTESIAN_POINT ( 'NONE',  ( -3.999999999999996447, -8.999999999999992895, 18.00000000000000000 ) ) ;
#21595=EDGE_LOOP ( 'NONE', ( #15742, #16297, #20674, #13684 ) ) ;
#21598=ADVANCED_FACE ( 'NONE', ( #24899 ), #3060, .T. ) ;
#21607=CARTESIAN_POINT ( 'NONE',  ( 1.878215178125004048, -5.746835883940462963, 0.3281249993854831737 ) ) ;
#21667=CARTESIAN_POINT ( 'NONE',  ( -1.878215178124998497, -12.25316411605951927, 3.140624999385482230 ) ) ;
#21693=ORIENTED_EDGE ( 'NONE', *, *, #5556, .T. ) ;
#21696=VERTEX_POINT ( 'NONE', #13762 ) ;
#21706=CARTESIAN_POINT ( 'NONE',  ( -3.756430356249997882, -11.16877607737301226, 2.203124999385479565 ) ) ;
#21707=CARTESIAN_POINT ( 'NONE',  ( 1.878215178125004048, -5.746835883940462963, 0.7781249993854856273 ) ) ;
#21713=CARTESIAN_POINT ( 'NONE',  ( -1.999999999999998224, -12.46410161513774639, 0.7500000000000006661 ) ) ;
#21715=CARTESIAN_POINT ( 'NONE',  ( 2.000000000000000888, -12.46410161513774817, 2.568749998770967213 ) ) ;
#21751=DIRECTION ( 'NONE',  ( 0.000000000000000000, 0.000000000000000000, 1.000000000000000000 ) ) ;
#21779=CARTESIAN_POINT ( 'NONE',  ( -1.999999999999998224, -12.46410161513774639, 1.143749998770968279 ) ) ;
#21785=CARTESIAN_POINT ( 'NONE',  ( 4.000000000000049738, -6.690598923241514839, 4.481249998770968190 ) ) ;
#21806=CARTESIAN_POINT ( 'NONE',  ( 3.756430356250003655, -8.999999999999992895, 2.840624999385484184 ) ) ;
#21829=CARTESIAN_POINT ( 'NONE',  ( 4.000000000000003553, -8.999999999999992895, 2.700000000000001066 ) ) ;
#21841=CARTESIAN_POINT ( 'NONE',  ( -1.878215178124995832, -5.746835883940462963, 3.890624999385482674 ) ) ;
#21842=CARTESIAN_POINT ( 'NONE',  ( 2.620986760973688460E-15, -13.61880215351699874, 3.431249998770965703 ) ) ;
#21848=CARTESIAN_POINT ( 'NONE',  ( 4.000000000000003553, -6.690598923241489970, 1.837499999999995914 ) ) ;
#21849=CARTESIAN_POINT ( 'NONE',  ( -3.999999999999996447, -8.999999999999992895, 1.125000000000000888 ) ) ;
#21874=CARTESIAN_POINT ( 'NONE',  ( -3.756430356249996994, -8.999999999999992895, 0.9281249993854829849 ) ) ;
#21880=CARTESIAN_POINT ( 'NONE',  ( -3.756430356249997438, -11.16877607737301048, 0.5156249993854836733 ) ) ;
#21888=ORIENTED_EDGE ( 'NONE', *, *, #10589, .F. ) ;
#21930=CARTESIAN_POINT ( 'NONE',  ( -3.756430356249996105, -6.831223922626973533, 4.378124999385480720 ) ) ;
#21932=AXIS2_PLACEMENT_3D ( 'NONE', #6280, #18693, #18192 ) ;
#21934=( LENGTH_UNIT ( ) NAMED_UNIT ( * ) SI_UNIT ( .MILLI., .METRE. ) );
#21936=DIRECTION ( 'NONE',  ( -0.000000000000000000, -0.000000000000000000, -1.000000000000000000 ) ) ;
#21939=CARTESIAN_POINT ( 'NONE',  ( 2.620986760973688460E-15, -13.61880215351699874, 2.081249998770966947 ) ) ;
#21956=VECTOR ( 'NONE', #798, 1000.000000000000000 ) ;
#21962=EDGE_CURVE ( 'NONE', #7351, #20735, #7914, .T. ) ;
#21966=CARTESIAN_POINT ( 'NONE',  ( -3.756430356249996994, -8.999999999999992895, 1.715624999385483074 ) ) ;
#21967=CARTESIAN_POINT ( 'NONE',  ( 4.000000000000003553, -6.690598923241489970, 3.131249998770965881 ) ) ;
#21995=DIRECTION ( 'NONE',  ( -0.000000000000000000, -0.000000000000000000, -1.000000000000000000 ) ) ;
#22003=DIRECTION ( 'NONE',  ( -0.000000000000000000, -0.000000000000000000, -1.000000000000000000 ) ) ;
#22048=CARTESIAN_POINT ( 'NONE',  ( -3.756430356249996994, -8.999999999999992895, 3.965624999385481519 ) ) ;
#22052=FILL_AREA_STYLE_COLOUR ( '', #12265 ) ;
#22058=CARTESIAN_POINT ( 'NONE',  ( -3.999999999999982681, -11.30940107675850292, 2.006249998770965437 ) ) ;
#22064=CARTESIAN_POINT ( 'NONE',  ( -3.999999999999949818, -6.690598923241462437, 2.437499999999999112 ) ) ;
#22066=DIRECTION ( 'NONE',  ( -0.000000000000000000, -0.000000000000000000, -1.000000000000000000 ) ) ;
#22085=CARTESIAN_POINT ( 'NONE',  ( 4.000000000000003553, -8.999999999999992895, 3.543749998770967302 ) ) ;
#22099=CARTESIAN_POINT ( 'NONE',  ( -3.999999999999996447, -8.999999999999992895, 1.574999999999999956 ) ) ;
#22120=CARTESIAN_POINT ( 'NONE',  ( 3.756430356250002323, -11.16877607737301226, 3.815624999385482052 ) ) ;
#22127=CARTESIAN_POINT ( 'NONE',  ( -1.878215178124995832, -5.746835883940462963, 0.7406249993854828739 ) ) ;
#22132=DIRECTION ( 'NONE',  ( 1.000000000000000000, 0.000000000000000000, 0.000000000000000000 ) ) ;
#22136=ADVANCED_FACE ( 'NONE', ( #8781 ), #20604, .T. ) ;
#22190=CARTESIAN_POINT ( 'NONE',  ( 1.878215178125000939, -12.25316411605952283, 3.665624999385483473 ) ) ;
#22194=CARTESIAN_POINT ( 'NONE',  ( 4.000000000000003553, -8.999999999999992895, 2.249999999999998668 ) ) ;
#22226=CARTESIAN_POINT ( 'NONE',  ( 2.000000000000000888, -12.46410161513774817, 4.818749998770965881 ) ) ;
#22259=CARTESIAN_POINT ( 'NONE',  ( 2.672651547586948120E-15, -13.33755215474602984, 3.290624999385483918 ) ) ;
#22266=CARTESIAN_POINT ( 'NONE',  ( 2.672651547586948120E-15, -13.33755215474602984, 2.278124999385481519 ) ) ;
#22269=CARTESIAN_POINT ( 'NONE',  ( -3.756430356249996105, -6.831223922626973533, 1.790624999385485028 ) ) ;
#22276=FACE_OUTER_BOUND ( 'NONE', #6874, .T. ) ;
#22293=( BOUNDED_CURVE ( )  B_SPLINE_CURVE ( 2, ( #1589, #19241, #15207, #20962, #21087, #17169, #13236 ),
 .UNSPECIFIED., .F., .F. ) 
 B_SPLINE_CURVE_WITH_KNOTS ( ( 3, 2, 2, 3 ),
 ( 0.7999999999999999334, 0.8166666666666665408, 0.8333333333333332593, 0.8499999999999998668 ),
 .UNSPECIFIED. ) 
 CURVE ( )  GEOMETRIC_REPRESENTATION_ITEM ( )  RATIONAL_B_SPLINE_CURVE ( ( 1.000000000000000888, 0.8660254037844378194, 1.000000000000000000, 0.8660254037844387076, 1.000000000000000000, 0.8660254037844395958, 0.9999999999999991118 ) ) 
 REPRESENTATION_ITEM ( '' )  );
#22333=CARTESIAN_POINT ( 'NONE',  ( 2.620986760973688460E-15, -13.61880215351699874, 1.237499999999996270 ) ) ;
#22347=CARTESIAN_POINT ( 'NONE',  ( -3.756430356249997882, -11.16877607737301226, 1.415624999385483029 ) ) ;
#22352=CARTESIAN_POINT ( 'NONE',  ( -3.999999999999996447, -8.999999999999992895, 3.824999999999998401 ) ) ;
#22377=CARTESIAN_POINT ( 'NONE',  ( 3.756430356250003655, -8.999999999999992895, 3.853124999385483473 ) ) ;
#22382=EDGE_CURVE ( 'NONE', #10226, #13593, #20435, .T. ) ;
#22384=CARTESIAN_POINT ( 'NONE',  ( -3.756430356249996994, -8.999999999999992895, 1.265624999385484006 ) ) ;
#22388=CARTESIAN_POINT ( 'NONE',  ( 1.878215178125004048, -5.746835883940462963, 1.678124999385483651 ) ) ;
#22414=EDGE_CURVE ( 'NONE', #15910, #23657, #11574, .T. ) ;
#22421=CARTESIAN_POINT ( 'NONE',  ( 2.000000000000000888, -12.46410161513774817, 0.3750000000000003331 ) ) ;
#22469=ORIENTED_EDGE ( 'NONE', *, *, #2307, .T. ) ;
#22477=CARTESIAN_POINT ( 'NONE',  ( -3.756430356249997882, -11.16877607737301226, 0.9656249993854834068 ) ) ;
#22481=CARTESIAN_POINT ( 'NONE',  ( 4.000000000000018652, -6.690598923241496188, 3.637499999999998401 ) ) ;
#22488=CARTESIAN_POINT ( 'NONE',  ( -1.999999999999995781, -5.535898384862237620, 2.849999999999998312 ) ) ;
#22511=CARTESIAN_POINT ( 'NONE',  ( 3.756430356250004099, -6.831223922626973533, 2.990624999385484539 ) ) ;
#22520=CARTESIAN_POINT ( 'NONE',  ( 3.756430356250003655, -8.999999999999992895, 2.840624999385484184 ) ) ;
#22522=CARTESIAN_POINT ( 'NONE',  ( 4.000000000000003553, -6.690598923241489970, 4.087499999999997691 ) ) ;
#22524=LINE ( 'NONE', #12195, #18860 ) ;
#22525=CARTESIAN_POINT ( 'NONE',  ( 2.672651547586948120E-15, -13.33755215474603162, 1.940624999385484939 ) ) ;
#22527=VERTEX_POINT ( 'NONE', #9234 ) ;
#22534=CARTESIAN_POINT ( 'NONE',  ( -1.999999999999995781, -5.535898384862237620, 2.343749998770968013 ) ) ;
#22540=ORIENTED_EDGE ( 'NONE', *, *, #5662, .T. ) ;
#22556=CARTESIAN_POINT ( 'NONE',  ( 2.000000000000000888, -12.46410161513774817, 2.174999999999999822 ) ) ;
#22567=FACE_OUTER_BOUND ( 'NONE', #23818, .T. ) ;
#22583=CARTESIAN_POINT ( 'NONE',  ( 4.000000000000003553, -8.999999999999992895, 0.9000000000000014655 ) ) ;
#22615=CARTESIAN_POINT ( 'NONE',  ( -1.999999999999998224, -12.46410161513774639, 3.393749998770966503 ) ) ;
#22617=CARTESIAN_POINT ( 'NONE',  ( 2.672651547586948120E-15, -13.33755215474602984, 2.390624999385484450 ) ) ;
#22627=DIRECTION ( 'NONE',  ( -0.000000000000000000, -0.000000000000000000, -1.000000000000000000 ) ) ;
#22645=ORIENTED_EDGE ( 'NONE', *, *, #2992, .T. ) ;
#22652=CARTESIAN_POINT ( 'NONE',  ( -3.756430356249996994, -8.999999999999992895, 2.278124999385483740 ) ) ;
#22656=DIRECTION ( 'NONE',  ( -1.000000000000000000, 0.000000000000000000, 0.000000000000000000 ) ) ;
#22657=ADVANCED_FACE ( 'NONE', ( #8017, #8403 ), #6049, .T. ) ;
#22660=CARTESIAN_POINT ( 'NONE',  ( 1.878215178125004048, -5.746835883940462963, 3.815624999385484273 ) ) ;
#22665=CARTESIAN_POINT ( 'NONE',  ( 3.735045420075836212E-15, -4.662447845253954171, 0.8156249993854834957 ) ) ;
#22708=CARTESIAN_POINT ( 'NONE',  ( -1.999999999999998224, -12.46410161513774639, 4.293749998770968190 ) ) ;
#22718=CARTESIAN_POINT ( 'NONE',  ( 3.999999999999954259, -6.690598923241460660, 0.9375000000000014433 ) ) ;
#22744=EDGE_LOOP ( 'NONE', ( #13624, #12701 ) ) ;
#22747=CARTESIAN_POINT ( 'NONE',  ( -2.999999999999996891, -8.999999999999992895, 0.000000000000000000 ) ) ;
#22748=CARTESIAN_POINT ( 'NONE',  ( 3.756430356250004099, -6.831223922626973533, 2.990624999385484539 ) ) ;
#22750=EDGE_CURVE ( 'NONE', #6676, #12847, #21287, .T. ) ;
#22779=CARTESIAN_POINT ( 'NONE',  ( 1.878215178125000939, -12.25316411605952283, 0.5156249993854833402 ) ) ;
#22785=CARTESIAN_POINT ( 'NONE',  ( 2.672651547586948120E-15, -13.33755215474602984, 4.528124999385480187 ) ) ;
#22786=CARTESIAN_POINT ( 'NONE',  ( 3.469446951953614189E-15, -8.999999999999992895, 18.00000000000000000 ) ) ;
#22787=CARTESIAN_POINT ( 'NONE',  ( 2.620986760973688460E-15, -13.61880215351699874, 4.387499999999998401 ) ) ;
#22790=CARTESIAN_POINT ( 'NONE',  ( 3.735045420075836212E-15, -4.662447845253954171, 2.615624999385482319 ) ) ;
#22824=CARTESIAN_POINT ( 'NONE',  ( 1.878215178125004048, -5.746835883940462963, 0.2156249993854816860 ) ) ;
#22868=CARTESIAN_POINT ( 'NONE',  ( 3.756430356250002323, -11.16877607737301226, 1.565624999385482941 ) ) ;
#22869=EDGE_CURVE ( 'NONE', #4035, #15232, #2731, .T. ) ;
#22872=CARTESIAN_POINT ( 'NONE',  ( -3.999999999999996447, -8.999999999999992895, 1.968749998770967569 ) ) ;
#22877=CARTESIAN_POINT ( 'NONE',  ( 3.878215178125003604, -8.999999999999992895, 0.07031249969274150358 ) ) ;
#22886=CARTESIAN_POINT ( 'NONE',  ( -3.999999999999996447, -8.999999999999992895, 2.925000000000000711 ) ) ;
#22899=CARTESIAN_POINT ( 'NONE',  ( -1.878215178124995832, -5.746835883940462963, 0.7406249993854828739 ) ) ;
#22906=CARTESIAN_POINT ( 'NONE',  ( -3.999999999999996447, -8.999999999999992895, 0.2249999999999995060 ) ) ;
#22908=CARTESIAN_POINT ( 'NONE',  ( -3.999999999999996447, -8.999999999999992895, 4.275000000000001243 ) ) ;
#22912=CARTESIAN_POINT ( 'NONE',  ( 1.878215178125004048, -5.746835883940462963, 3.928124999385485872 ) ) ;
#22978=( BOUNDED_SURFACE ( )  B_SPLINE_SURFACE ( 1, 2, ( 
 ( #14852, #988, #22824, #19023, #9081, #24647, #17065, #10648, #14726, #12877, #20854, #10220, #176, #12443, #18217, #10337, #22127, #20029, #8653, #20410, #689, #16126, #298, #2384, #18098, #24088, #10097, #24220, #8269, #16634, #22384, #18338, #18602, #14540, #6307, #14679, #14159, #6438, #434, #8147, #4077, #4214, #6171, #16392, #2134, #16251, #10480, #24360, #12050, #10611, #2512, #18479, #20289, #12580, #14423, #12193, #14301, #22266, #6686, #4345, #2264, #568, #20163, #12321, #24603, #4598, #8404, #8538, #4466, #16519, #24480, #6559, #22520, #20560, #2649, #12718, #1332, #13109, #19230, #8787, #18863, #20954, #10730, #16776, #2769, #16909, #951, #9308, #15069, #11006, #11249, #7216, #24874, #7339, #6829, #24992, #3037, #18716, #22660, #14811, #808, #9044, #17293, #7079, #20686, #19103, #12837, #17026, #23044, #6953, #25259, #5130, #4992, #18985, #4748, #24744, #12970, #22785, #21080, #1188, #9169 ),
 ( #8929, #3275, #17159, #25131, #14932, #4861, #22906, #13227, #10862, #1070, #20812, #2895, #3156, #11125, #15199, #23168, #5248, #21198, #11514, #3411, #21713, #13496, #15827, #15317, #23285, #7459, #13735, #21580, #9813, #11390, #23801, #3660, #15449, #15708, #19365, #25643, #1967, #1717, #19483, #23672, #9430, #9691, #5369, #17675, #13360, #5889, #5634, #21332, #1578, #21848, #19754, #17796, #9549, #9931, #17538, #13873, #3541, #25511, #1459, #23419, #3797, #7724, #5749, #1851, #21466, #17917, #7599, #17412, #11776, #15584, #3930, #25375, #5506, #23553, #25762, #11637, #7843, #13614, #11899, #19613, #19867, #9, #14681, #8539, #14813, #3039, #2651, #6688, #24877, #16636, #6955, #18339, #18604, #2771, #16393, #4600, #24746, #12720, #435, #14935, #811, #6831, #8655, #953, #4750, #4468, #6561, #14542, #20957, #22522, #16521, #16778, #12444, #24481, #22908, #18865, #20411, #22787, #8405, #12582, #14424 ) ),
 .UNSPECIFIED., .F., .F., .F. ) 
 B_SPLINE_SURFACE_WITH_KNOTS ( ( 2, 2 ),
 ( 3, 2, 2, 2, 2, 2, 2, 2, 2, 2, 2, 2, 2, 2, 2, 2, 2, 2, 2, 2, 2, 2, 2, 2, 2, 2, 2, 2, 2, 2, 2, 2, 2, 2, 2, 2, 2, 2, 2, 2, 2, 2, 2, 2, 2, 2, 2, 2, 2, 2, 2, 2, 2, 2, 2, 2, 2, 2, 2, 2, 3 ),
 ( 0.000000000000000000, 1.000000000000000000 ),
 ( 0.000000000000000000, 0.01666666666666666644, 0.03333333333333333287, 0.05000000000000000278, 0.06666666666666666574, 0.08333333333333332871, 0.1000000000000000056, 0.1166666666666666685, 0.1333333333333333315, 0.1499999999999999944, 0.1666666666666666574, 0.1833333333333333204, 0.2000000000000000111, 0.2166666666666666741, 0.2333333333333333370, 0.2500000000000000000, 0.2666666666666666630, 0.2833333333333333259, 0.2999999999999999889, 0.3166666666666666519, 0.3333333333333333148, 0.3499999999999999778, 0.3666666666666666408, 0.3833333333333333592, 0.4000000000000000222, 0.4166666666666666852, 0.4333333333333333481, 0.4500000000000000111, 0.4666666666666666741, 0.4833333333333333370, 0.5000000000000000000, 0.5166666666666667185, 0.5333333333333333259, 0.5500000000000000444, 0.5666666666666666519, 0.5833333333333333703, 0.5999999999999999778, 0.6166666666666666963, 0.6333333333333333037, 0.6500000000000000222, 0.6666666666666666297, 0.6833333333333333481, 0.6999999999999999556, 0.7166666666666666741, 0.7333333333333332815, 0.7500000000000000000, 0.7666666666666667185, 0.7833333333333333259, 0.8000000000000000444, 0.8166666666666666519, 0.8333333333333333703, 0.8499999999999999778, 0.8666666666666666963, 0.8833333333333333037, 0.9000000000000000222, 0.9166666666666666297, 0.9333333333333333481, 0.9499999999999999556, 0.9666666666666666741, 0.9833333333333332815, 1.000000000000000000 ),
 .UNSPECIFIED. ) 
 GEOMETRIC_REPRESENTATION_ITEM ( )  RATIONAL_B_SPLINE_SURFACE ( (
 ( 1.000000000000000000, 0.8660254037844387076, 1.000000000000000000, 0.8660254037844387076, 1.000000000000000000, 0.8660254037844387076, 1.000000000000000000, 0.8660254037844387076, 1.000000000000000000, 0.8660254037844387076, 1.000000000000000000, 0.8660254037844387076, 1.000000000000000000, 0.8660254037844387076, 1.000000000000000000, 0.8660254037844387076, 1.000000000000000000, 0.8660254037844387076, 1.000000000000000000, 0.8660254037844387076, 1.000000000000000000, 0.8660254037844387076, 1.000000000000000000, 0.8660254037844387076, 1.000000000000000000, 0.8660254037844387076, 1.000000000000000000, 0.8660254037844387076, 1.000000000000000000, 0.8660254037844387076, 1.000000000000000000, 0.8660254037844387076, 1.000000000000000000, 0.8660254037844387076, 1.000000000000000000, 0.8660254037844387076, 1.000000000000000000, 0.8660254037844387076, 1.000000000000000000, 0.8660254037844387076, 1.000000000000000000, 0.8660254037844387076, 1.000000000000000000, 0.8660254037844387076, 1.000000000000000000, 0.8660254037844387076, 1.000000000000000000, 0.8660254037844387076, 1.000000000000000000, 0.8660254037844387076, 1.000000000000000000, 0.8660254037844387076, 1.000000000000000000, 0.8660254037844387076, 1.000000000000000000, 0.8660254037844387076, 1.000000000000000000, 0.8660254037844387076, 1.000000000000000000, 0.8660254037844387076, 1.000000000000000000, 0.8660254037844387076, 1.000000000000000000, 0.8660254037844387076, 1.000000000000000000, 0.8660254037844387076, 1.000000000000000000, 0.8660254037844387076, 1.000000000000000000, 0.8660254037844387076, 1.000000000000000000, 0.8660254037844387076, 1.000000000000000000, 0.8660254037844387076, 1.000000000000000000, 0.8660254037844387076, 1.000000000000000000, 0.8660254037844387076, 1.000000000000000000, 0.8660254037844387076, 1.000000000000000000, 0.8660254037844387076, 1.000000000000000000, 0.8660254037844387076, 1.000000000000000000, 0.8660254037844387076, 1.000000000000000000, 0.8660254037844387076, 1.000000000000000000, 0.8660254037844387076, 1.000000000000000000, 0.8660254037844387076, 1.000000000000000000, 0.8660254037844387076, 1.000000000000000000, 0.8660254037844387076, 1.000000000000000000, 0.8660254037844387076, 1.000000000000000000, 0.8660254037844387076, 1.000000000000000000, 0.8660254037844387076, 1.000000000000000000, 0.8660254037844387076, 1.000000000000000000, 0.8660254037844387076, 1.000000000000000000, 0.8660254037844387076, 1.000000000000000000, 0.8660254037844387076, 1.000000000000000000, 0.8660254037844387076, 1.000000000000000000, 0.8660254037844387076, 1.000000000000000000, 0.8660254037844387076, 1.000000000000000000, 0.8660254037844387076, 1.000000000000000000, 0.8660254037844387076, 1.000000000000000000),
 ( 1.000000000000000000, 0.8660254037844387076, 1.000000000000000000, 0.8660254037844387076, 1.000000000000000000, 0.8660254037844387076, 1.000000000000000000, 0.8660254037844387076, 1.000000000000000000, 0.8660254037844387076, 1.000000000000000000, 0.8660254037844387076, 1.000000000000000000, 0.8660254037844387076, 1.000000000000000000, 0.8660254037844387076, 1.000000000000000000, 0.8660254037844387076, 1.000000000000000000, 0.8660254037844387076, 1.000000000000000000, 0.8660254037844387076, 1.000000000000000000, 0.8660254037844387076, 1.000000000000000000, 0.8660254037844387076, 1.000000000000000000, 0.8660254037844387076, 1.000000000000000000, 0.8660254037844387076, 1.000000000000000000, 0.8660254037844387076, 1.000000000000000000, 0.8660254037844387076, 1.000000000000000000, 0.8660254037844387076, 1.000000000000000000, 0.8660254037844387076, 1.000000000000000000, 0.8660254037844387076, 1.000000000000000000, 0.8660254037844387076, 1.000000000000000000, 0.8660254037844387076, 1.000000000000000000, 0.8660254037844387076, 1.000000000000000000, 0.8660254037844387076, 1.000000000000000000, 0.8660254037844387076, 1.000000000000000000, 0.8660254037844387076, 1.000000000000000000, 0.8660254037844387076, 1.000000000000000000, 0.8660254037844387076, 1.000000000000000000, 0.8660254037844387076, 1.000000000000000000, 0.8660254037844387076, 1.000000000000000000, 0.8660254037844387076, 1.000000000000000000, 0.8660254037844387076, 1.000000000000000000, 0.8660254037844387076, 1.000000000000000000, 0.8660254037844387076, 1.000000000000000000, 0.8660254037844387076, 1.000000000000000000, 0.8660254037844387076, 1.000000000000000000, 0.8660254037844387076, 1.000000000000000000, 0.8660254037844387076, 1.000000000000000000, 0.8660254037844387076, 1.000000000000000000, 0.8660254037844387076, 1.000000000000000000, 0.8660254037844387076, 1.000000000000000000, 0.8660254037844387076, 1.000000000000000000, 0.8660254037844387076, 1.000000000000000000, 0.8660254037844387076, 1.000000000000000000, 0.8660254037844387076, 1.000000000000000000, 0.8660254037844387076, 1.000000000000000000, 0.8660254037844387076, 1.000000000000000000, 0.8660254037844387076, 1.000000000000000000, 0.8660254037844387076, 1.000000000000000000, 0.8660254037844387076, 1.000000000000000000, 0.8660254037844387076, 1.000000000000000000, 0.8660254037844387076, 1.000000000000000000, 0.8660254037844387076, 1.000000000000000000, 0.8660254037844387076, 1.000000000000000000, 0.8660254037844387076, 1.000000000000000000, 0.8660254037844387076, 1.000000000000000000, 0.8660254037844387076, 1.000000000000000000, 0.8660254037844387076, 1.000000000000000000, 0.8660254037844387076, 1.000000000000000000, 0.8660254037844387076, 1.000000000000000000) ) ) 
 REPRESENTATION_ITEM ( '' )  SURFACE ( )  );
#23000=CARTESIAN_POINT ( 'NONE',  ( -3.756430356249996105, -6.831223922626973533, 1.228124999385478144 ) ) ;
#23002=CARTESIAN_POINT ( 'NONE',  ( 1.878215178125000939, -12.25316411605952283, 4.678124999385483207 ) ) ;
#23032=ORIENTED_EDGE ( 'NONE', *, *, #18300, .T. ) ;
#23037=CARTESIAN_POINT ( 'NONE',  ( -3.756430356249996994, -8.999999999999992895, 1.265624999385484006 ) ) ;
#23038=CARTESIAN_POINT ( 'NONE',  ( 2.620986760973688460E-15, -13.61880215351699874, 2.531249998770966236 ) ) ;
#23044=CARTESIAN_POINT ( 'NONE',  ( 3.756430356250003655, -8.999999999999992895, 4.190624999385480720 ) ) ;
#23049=CARTESIAN_POINT ( 'NONE',  ( 3.735045420075836212E-15, -4.662447845253954171, 3.515624999385486227 ) ) ;
#23123=EDGE_LOOP ( 'NONE', ( #12884, #20228, #25840, #9824 ) ) ;
#23132=CARTESIAN_POINT ( 'NONE',  ( 3.756430356250003211, -6.831223922626973533, 1.528124999385481964 ) ) ;
#23138=CARTESIAN_POINT ( 'NONE',  ( 4.000000000000003553, -8.999999999999992895, 0.9000000000000014655 ) ) ;
#23162=CARTESIAN_POINT ( 'NONE',  ( 3.756430356250004099, -6.831223922626973533, 4.340624999385483740 ) ) ;
#23163=CARTESIAN_POINT ( 'NONE',  ( -1.999999999999998224, -12.46410161513774639, 2.493749998770968812 ) ) ;
#23168=CARTESIAN_POINT ( 'NONE',  ( 3.752267015613588906E-15, -4.381197846482986158, 0.5624999999999986677 ) ) ;
#23173=CARTESIAN_POINT ( 'NONE',  ( -3.999999999999982681, -6.690598923241479312, 0.5812499987709673910 ) ) ;
#23246=CARTESIAN_POINT ( 'NONE',  ( 3.756430356250003655, -8.999999999999992895, 1.940624999385482496 ) ) ;
#23247=CARTESIAN_POINT ( 'NONE',  ( 3.756430356250003655, -8.999999999999992895, 4.753124999385485161 ) ) ;
#23260=EDGE_CURVE ( 'NONE', #19181, #3646, #4252, .T. ) ;
#23262=CARTESIAN_POINT ( 'NONE',  ( 4.000000000000003553, -8.999999999999992895, 4.500000000000000888 ) ) ;
#23268=ORIENTED_EDGE ( 'NONE', *, *, #8390, .F. ) ;
#23280=CARTESIAN_POINT ( 'NONE',  ( 3.756430356250003655, -8.999999999999992895, 0.5906249993854819635 ) ) ;
#23281=CARTESIAN_POINT ( 'NONE',  ( 4.000000000000001776, -11.30940107675849760, 2.606249998770964194 ) ) ;
#23285=CARTESIAN_POINT ( 'NONE',  ( 4.000000000000003553, -8.999999999999992895, 0.9000000000000014655 ) ) ;
#23358=FACE_OUTER_BOUND ( 'NONE', #13946, .T. ) ;
#23376=CARTESIAN_POINT ( 'NONE',  ( 1.878215178125004048, -5.746835883940462963, 0.6656249993854841396 ) ) ;
#23379=CARTESIAN_POINT ( 'NONE',  ( -1.878215178124995832, -5.746835883940462963, 3.553124999385485427 ) ) ;
#23393=CARTESIAN_POINT ( 'NONE',  ( 3.878215178125003604, -8.999999999999992895, 4.823437499078226942 ) ) ;
#23394=CARTESIAN_POINT ( 'NONE',  ( -3.999999999999936051, -11.30940107675852779, 4.312500000000001776 ) ) ;
#23413=CARTESIAN_POINT ( 'NONE',  ( -3.756430356249997882, -11.16877607737301226, 3.553124999385482763 ) ) ;
#23414=CARTESIAN_POINT ( 'NONE',  ( -3.999999999999996447, -8.999999999999992895, 1.518749998770968501 ) ) ;
#23419=CARTESIAN_POINT ( 'NONE',  ( 4.000000000000001776, -11.30940107675849760, 2.212499999999997691 ) ) ;
#23425=CARTESIAN_POINT ( 'NONE',  ( -1.878215178124998497, -12.25316411605951927, 4.603124999385483918 ) ) ;
#23427=CARTESIAN_POINT ( 'NONE',  ( -1.999999999999998224, -12.46410161513774639, 4.743749998770967480 ) ) ;
#23433=EDGE_LOOP ( 'NONE', ( #12300, #13812, #1792, #6037 ) ) ;
#23466=ORIENTED_EDGE ( 'NONE', *, *, #1688, .T. ) ;
#23469=CARTESIAN_POINT ( 'NONE',  ( -3.999999999999996447, -8.999999999999992895, 4.668749998770968190 ) ) ;
#23512=CARTESIAN_POINT ( 'NONE',  ( 3.735045420075836212E-15, -4.662447845253954171, 4.415624999385481253 ) ) ;
#23545=CARTESIAN_POINT ( 'NONE',  ( 3.756430356250003655, -8.999999999999992895, 3.740624999385481875 ) ) ;
#23546=CARTESIAN_POINT ( 'NONE',  ( 4.000000000000003553, -8.999999999999992895, 0.8437499987709664584 ) ) ;
#23553=CARTESIAN_POINT ( 'NONE',  ( 4.000000000000003553, -6.690598923241489970, 2.737499999999999378 ) ) ;
#23571=EDGE_LOOP ( 'NONE', ( #17816, #25417, #9052, #6567 ) ) ;
#23583=CARTESIAN_POINT ( 'NONE',  ( -3.756430356249996105, -6.831223922626973533, 0.4406249993854816638 ) ) ;
#23599=CARTESIAN_POINT ( 'NONE',  ( 2.000000000000003997, -5.535898384862238508, 4.125000000000000000 ) ) ;
#23613=EDGE_CURVE ( 'NONE', #13776, #15232, #23901, .T. ) ;
#23635=CARTESIAN_POINT ( 'NONE',  ( 1.878215178125000939, -12.25316411605952283, 2.765624999385481786 ) ) ;
#23643=FACE_OUTER_BOUND ( 'NONE', #3195, .T. ) ;
#23645=VERTEX_POINT ( 'NONE', #20876 ) ;
#23653=CARTESIAN_POINT ( 'NONE',  ( -4.000000000000043521, -11.30940107675846562, 2.512500000000000622 ) ) ;
#23657=VERTEX_POINT ( 'NONE', #6370 ) ;
#23667=CARTESIAN_POINT ( 'NONE',  ( 1.878215178125004048, -5.746835883940462963, 3.365624999385481875 ) ) ;
#23668=CARTESIAN_POINT ( 'NONE',  ( 4.000000000000001776, -11.30940107675849760, 3.506249998770968102 ) ) ;
#23672=CARTESIAN_POINT ( 'NONE',  ( 3.752267015613588906E-15, -4.381197846482986158, 1.462499999999998135 ) ) ;
#23674=CARTESIAN_POINT ( 'NONE',  ( -4.000000000000021316, -11.30940107675847806, 2.456249998770964282 ) ) ;
#23694=CARTESIAN_POINT ( 'NONE',  ( -3.756430356249996994, -8.999999999999992895, 1.378124999385485605 ) ) ;
#23735=CARTESIAN_POINT ( 'NONE',  ( 2.620986760973688460E-15, -13.61880215351699874, 2.981249998770965970 ) ) ;
#23747=CARTESIAN_POINT ( 'NONE',  ( -3.999999999999996447, -8.999999999999992895, 1.968749998770967569 ) ) ;
#23755=CARTESIAN_POINT ( 'NONE',  ( -1.878215178124995832, -5.746835883940462963, 3.890624999385482674 ) ) ;
#23765=CARTESIAN_POINT ( 'NONE',  ( 2.000000000000000888, -12.46410161513774817, 2.118749998770968368 ) ) ;
#23775=ORIENTED_EDGE ( 'NONE', *, *, #18928, .F. ) ;
#23793=CARTESIAN_POINT ( 'NONE',  ( 1.878215178125000939, -12.25316411605952283, 2.765624999385481786 ) ) ;
#23794=CARTESIAN_POINT ( 'NONE',  ( 2.000000000000000888, -12.46410161513774817, 3.918749998770967746 ) ) ;
#23801=CARTESIAN_POINT ( 'NONE',  ( -3.999999999999996447, -8.999999999999992895, 1.125000000000000888 ) ) ;
#23818=EDGE_LOOP ( 'NONE', ( #10424, #5353, #12878, #17692, #10236, #20301, #9468, #2142, #15416, #10650, #8613, #16786, #13597, #8951, #24728, #2332, #20936, #12400, #2945, #3648, #15158, #20467, #7965 ) ) ;
#23827=CARTESIAN_POINT ( 'NONE',  ( -1.878215178124998497, -12.25316411605951927, 1.003124999385485161 ) ) ;
#23837=CARTESIAN_POINT ( 'NONE',  ( 3.756430356250003655, -8.999999999999992895, 0.7031249993854835623 ) ) ;
#23855=AXIS2_PLACEMENT_3D ( 'NONE', #6234, #21936, #25729 ) ;
#23896=CARTESIAN_POINT ( 'NONE',  ( 1.878215178125000939, -12.25316411605952283, 3.215624999385484184 ) ) ;
#23901=LINE ( 'NONE', #12120, #4238 ) ;
#23908=ORIENTED_EDGE ( 'NONE', *, *, #19511, .T. ) ;
#23930=CIRCLE ( 'NONE', #9322, 3.000000000000000444 ) ;
#23931=CARTESIAN_POINT ( 'NONE',  ( 2.672651547586948120E-15, -13.33755215474602984, 1.828124999385481786 ) ) ;
#23932=CARTESIAN_POINT ( 'NONE',  ( -3.999999999999997335, -11.30940107675849404, 3.806249998770963927 ) ) ;
#23935=CARTESIAN_POINT ( 'NONE',  ( 4.000000000000032863, -11.30940107675847983, 1.706249998770969389 ) ) ;
#23964=CARTESIAN_POINT ( 'NONE',  ( -1.878215178124998497, -12.25316411605951927, 1.453124999385484228 ) ) ;
#24012=CYLINDRICAL_SURFACE ( 'NONE', #5032, 4.000000000000000000 ) ;
#24019=CARTESIAN_POINT ( 'NONE',  ( 2.672651547586948120E-15, -13.33755215474603162, 3.628124999385485161 ) ) ;
#24021=VECTOR ( 'NONE', #21303, 999.9999999999998863 ) ;
#24051=CARTESIAN_POINT ( 'NONE',  ( -3.756430356249996994, -8.999999999999992895, 4.415624999385483918 ) ) ;
#24052=CARTESIAN_POINT ( 'NONE',  ( -3.999999999999996003, -6.690598923241487306, 4.181249998770965703 ) ) ;
#24061=CARTESIAN_POINT ( 'NONE',  ( 4.000000000000003553, -8.999999999999992895, 0.8437499987709664584 ) ) ;
#24079=FACE_OUTER_BOUND ( 'NONE', #1108, .T. ) ;
#24082=CARTESIAN_POINT ( 'NONE',  ( -1.878215178124998497, -12.25316411605951927, 1.903124999385483296 ) ) ;
#24086=EDGE_CURVE ( 'NONE', #702, #7351, #14281, .T. ) ;
#24088=CARTESIAN_POINT ( 'NONE',  ( 3.756430356250004099, -6.831223922626973533, 1.078124999385482452 ) ) ;
#24091=CARTESIAN_POINT ( 'NONE',  ( -1.999999999999998224, -12.46410161513774639, 3.449999999999998401 ) ) ;
#24115=CARTESIAN_POINT ( 'NONE',  ( 4.000000000000051514, -11.30940107675846917, 1.256249998770965881 ) ) ;
#24138=CARTESIAN_POINT ( 'NONE',  ( -1.878215178124998497, -12.25316411605951927, 3.590624999385481075 ) ) ;
#24154=CARTESIAN_POINT ( 'NONE',  ( -3.999999999999996447, -8.999999999999992895, 2.474999999999997868 ) ) ;
#24155=VERTEX_POINT ( 'NONE', #8051 ) ;
#24175=AXIS2_PLACEMENT_3D ( 'NONE', #13583, #18159, #25610 ) ;
#24179=CARTESIAN_POINT ( 'NONE',  ( 2.672651547586948120E-15, -13.33755215474602984, 0.5906249993854855163 ) ) ;
#24214=CARTESIAN_POINT ( 'NONE',  ( 1.878215178125000939, -12.25316411605952283, 1.528124999385482852 ) ) ;
#24220=CARTESIAN_POINT ( 'NONE',  ( 3.735045420075836212E-15, -4.662447845253954171, 1.153124999385480187 ) ) ;
#24224=CARTESIAN_POINT ( 'NONE',  ( -3.756430356249996105, -6.831223922626973533, 1.340624999385481075 ) ) ;
#24298=CARTESIAN_POINT ( 'NONE',  ( -3.999999999999996447, -8.999999999999992895, 0.2249999999999995060 ) ) ;
#24319=CARTESIAN_POINT ( 'NONE',  ( -1.878215178124995832, -5.746835883940462963, 3.103124999385483029 ) ) ;
#24352=CARTESIAN_POINT ( 'NONE',  ( 3.756430356250003655, -8.999999999999992895, 1.603124999385485028 ) ) ;
#24353=CARTESIAN_POINT ( 'NONE',  ( -3.999999999999996447, -8.999999999999992895, 1.518749998770968501 ) ) ;
#24360=CARTESIAN_POINT ( 'NONE',  ( 3.756430356250002323, -11.16877607737301226, 1.903124999385483740 ) ) ;
#24366=CARTESIAN_POINT ( 'NONE',  ( 1.878215178125000939, -12.25316411605952283, 2.878124999385483385 ) ) ;
#24376=CARTESIAN_POINT ( 'NONE',  ( 4.000000000000003553, -8.999999999999992895, 2.193749998770967213 ) ) ;
#24385=LINE ( 'NONE', #8814, #20945 ) ;
#24408=EDGE_LOOP ( 'NONE', ( #14430, #22540, #705, #6119 ) ) ;
#24444=CARTESIAN_POINT ( 'NONE',  ( -3.756430356249996994, -8.999999999999992895, 0.9281249993854829849 ) ) ;
#24446=CYLINDRICAL_SURFACE ( 'NONE', #3437, 4.000000000000000000 ) ;
#24475=CARTESIAN_POINT ( 'NONE',  ( -1.878215178124998497, -12.25316411605951927, 2.803124999385484539 ) ) ;
#24476=CARTESIAN_POINT ( 'NONE',  ( -1.999999999999998224, -12.46410161513774639, 0.6937499987709692117 ) ) ;
#24480=CARTESIAN_POINT ( 'NONE',  ( 1.878215178125000939, -12.25316411605952283, 2.765624999385481786 ) ) ;
#24481=CARTESIAN_POINT ( 'NONE',  ( -3.999999999999996003, -6.690598923241487306, 4.237499999999998046 ) ) ;
#24484=CARTESIAN_POINT ( 'NONE',  ( -3.756430356249996105, -6.831223922626973533, 2.240624999385484539 ) ) ;
#24493=CARTESIAN_POINT ( 'NONE',  ( 2.000000000000003997, -5.535898384862238508, 2.268749998770969167 ) ) ;
#24495=ORIENTED_EDGE ( 'NONE', *, *, #14830, .T. ) ;
#24542=DIRECTION ( 'NONE',  ( -1.000000000000000000, 0.000000000000000000, 0.000000000000000000 ) ) ;
#24549=DIRECTION ( 'NONE',  ( -0.000000000000000000, -0.000000000000000000, -1.000000000000000000 ) ) ;
#24560=CARTESIAN_POINT ( 'NONE',  ( -3.756430356249995661, -6.831223922626973533, 2.240624999385484539 ) ) ;
#24581=CIRCLE ( 'NONE', #16659, 3.000000000000000444 ) ;
#24594=CARTESIAN_POINT ( 'NONE',  ( 2.672651547586948120E-15, -13.33755215474602984, 2.390624999385484450 ) ) ;
#24603=CARTESIAN_POINT ( 'NONE',  ( -1.878215178124995832, -5.746835883940462963, 2.540624999385482141 ) ) ;
#24608=CARTESIAN_POINT ( 'NONE',  ( 3.756430356250003211, -6.831223922626973533, 1.190624999385485383 ) ) ;
#24636=CARTESIAN_POINT ( 'NONE',  ( 4.000000000000003553, -8.999999999999992895, 2.249999999999998668 ) ) ;
#24641=CARTESIAN_POINT ( 'NONE',  ( 2.620986760973688460E-15, -13.61880215351699874, 0.3375000000000007438 ) ) ;
#24647=CARTESIAN_POINT ( 'NONE',  ( -3.756430356249995661, -6.831223922626973533, 0.3281249993854827851 ) ) ;
#24651=( BOUNDED_CURVE ( )  B_SPLINE_CURVE ( 2, ( #13590, #1689, #15802, #9663, #2070, #22064, #24154 ),
 .UNSPECIFIED., .F., .T. ) 
 B_SPLINE_CURVE_WITH_KNOTS ( ( 3, 2, 2, 3 ),
 ( 0.4999999999999997780, 0.5166666666666664964, 0.5333333333333329929, 0.5499999999999997113 ),
 .UNSPECIFIED. ) 
 CURVE ( )  GEOMETRIC_REPRESENTATION_ITEM ( )  RATIONAL_B_SPLINE_CURVE ( ( 1.000000000000001776, 0.8660254037844369313, 1.000000000000000000, 0.8660254037844387076, 1.000000000000000000, 0.8660254037844413721, 0.9999999999999973355 ) ) 
 REPRESENTATION_ITEM ( '' )  );
#24661=CARTESIAN_POINT ( 'NONE',  ( -1.878215178124998497, -12.25316411605951927, 4.490624999385482319 ) ) ;
#24691=FACE_OUTER_BOUND ( 'NONE', #23433, .T. ) ;
#24703=CARTESIAN_POINT ( 'NONE',  ( 1.878215178125004048, -5.746835883940462963, 2.128124999385486049 ) ) ;
#24728=ORIENTED_EDGE ( 'NONE', *, *, #9136, .T. ) ;
#24738=CARTESIAN_POINT ( 'NONE',  ( 2.672651547586948120E-15, -13.33755215474602984, 0.4781249993854826963 ) ) ;
#24744=CARTESIAN_POINT ( 'NONE',  ( -3.756430356249997882, -11.16877607737301226, 4.453124999385482674 ) ) ;
#24746=CARTESIAN_POINT ( 'NONE',  ( 4.000000000000003553, -8.999999999999992895, 3.599999999999999201 ) ) ;
#24750=CARTESIAN_POINT ( 'NONE',  ( 1.878215178125004048, -5.746835883940462963, 2.128124999385486049 ) ) ;
#24760=LINE ( 'NONE', #25273, #25831 ) ;
#24779=CARTESIAN_POINT ( 'NONE',  ( 4.000000000000003553, -8.999999999999992895, 4.893749998770967835 ) ) ;
#24802=CARTESIAN_POINT ( 'NONE',  ( 2.000000000000003997, -5.535898384862238508, 3.224999999999998757 ) ) ;
#24812=CARTESIAN_POINT ( 'NONE',  ( -3.999999999999996447, -8.999999999999992895, 18.00000000000000000 ) ) ;
#24813=( BOUNDED_CURVE ( )  B_SPLINE_CURVE ( 2, ( #16214, #12290, #5888, #8238, #10190, #23935, #8 ),
 .UNSPECIFIED., .F., .F. ) 
 B_SPLINE_CURVE_WITH_KNOTS ( ( 3, 2, 2, 3 ),
 ( 0.2500000000000002776, 0.2666666666666669405, 0.2833333333333335480, 0.3000000000000002109 ),
 .UNSPECIFIED. ) 
 CURVE ( )  GEOMETRIC_REPRESENTATION_ITEM ( )  RATIONAL_B_SPLINE_CURVE ( ( 0.9999999999999977796, 0.8660254037844409281, 1.000000000000000000, 0.8660254037844387076, 1.000000000000000000, 0.8660254037844369313, 1.000000000000001776 ) ) 
 REPRESENTATION_ITEM ( '' )  );
#24816=( GEOMETRIC_REPRESENTATION_CONTEXT ( 3 ) GLOBAL_UNCERTAINTY_ASSIGNED_CONTEXT ( ( #4955 ) ) GLOBAL_UNIT_ASSIGNED_CONTEXT ( ( #21934, #6103, #8201 ) ) REPRESENTATION_CONTEXT ( 'NONE', 'WORKASPACE' ) );
#24836=CARTESIAN_POINT ( 'NONE',  ( 1.878215178125000939, -12.25316411605952283, 2.878124999385483385 ) ) ;
#24839=CARTESIAN_POINT ( 'NONE',  ( 3.999999999999972466, -6.690598923241471319, 1.781249998770967125 ) ) ;
#24841=UNCERTAINTY_MEASURE_WITH_UNIT (LENGTH_MEASURE( 1.000000000000000082E-05 ), #15539, 'distance_accuracy_value', 'NONE');
#24842=PRODUCT_DEFINITION_CONTEXT ( 'detailed design', #20643, 'design' ) ;
#24859=ORIENTED_EDGE ( 'NONE', *, *, #22414, .F. ) ;
#24867=CARTESIAN_POINT ( 'NONE',  ( 3.756430356250004099, -6.831223922626973533, 0.6281249993854786107 ) ) ;
#24872=CARTESIAN_POINT ( 'NONE',  ( 4.000000000000003553, -8.999999999999992895, 0.4499999999999990119 ) ) ;
#24874=CARTESIAN_POINT ( 'NONE',  ( -1.878215178124998497, -12.25316411605951927, 3.590624999385481075 ) ) ;
#24877=CARTESIAN_POINT ( 'NONE',  ( -1.999999999999995781, -5.535898384862237620, 3.300000000000000711 ) ) ;
#24879=CARTESIAN_POINT ( 'NONE',  ( 3.756430356250003655, -8.999999999999992895, 3.403124999385484628 ) ) ;
#24887=ORIENTED_EDGE ( 'NONE', *, *, #16972, .T. ) ;
#24899=FACE_OUTER_BOUND ( 'NONE', #21595, .T. ) ;
#24959=CARTESIAN_POINT ( 'NONE',  ( -1.999999999999995781, -5.535898384862237620, 1.893749998770968723 ) ) ;
#24960=CARTESIAN_POINT ( 'NONE',  ( 3.752267015613588906E-15, -4.381197846482986158, 3.712500000000000355 ) ) ;
#24982=CYLINDRICAL_SURFACE ( 'NONE', #21125, 4.000000000000000000 ) ;
#24986=CARTESIAN_POINT ( 'NONE',  ( -3.756430356249995661, -6.831223922626973533, 0.7781249993854825187 ) ) ;
#24988=CARTESIAN_POINT ( 'NONE',  ( 4.000000000000003553, -8.999999999999992895, 2.643749998770966059 ) ) ;
#24992=CARTESIAN_POINT ( 'NONE',  ( 3.756430356250002323, -11.16877607737301226, 3.703124999385482674 ) ) ;
#24994=FACE_OUTER_BOUND ( 'NONE', #25076, .T. ) ;
#24998=CARTESIAN_POINT ( 'NONE',  ( 2.672651547586948120E-15, -13.33755215474603162, 4.640624999385483562 ) ) ;
#25006=EDGE_LOOP ( 'NONE', ( #24859, #856, #1201, #13894 ) ) ;
#25010=ORIENTED_EDGE ( 'NONE', *, *, #19431, .T. ) ;
#25027=VECTOR ( 'NONE', #6123, 1000.000000000000000 ) ;
#25056=DIRECTION ( 'NONE',  ( -0.000000000000000000, -0.000000000000000000, -1.000000000000000000 ) ) ;
#25068=( BOUNDED_CURVE ( )  B_SPLINE_CURVE ( 2, ( #15866, #13910, #17707, #14162, #1756, #23583, #5784, #21880, #13771, #3832, #11811, #3964, #23837, #11929, #19898, #22665, #20415, #2516, #10736, #4605, #439, #4348, #10615, #14306, #16640, #24608, #8409, #10485, #8272, #24224, #14545, #18485, #573, #8543, #16524, #4471, #12446, #18608, #22388, #6311, #10341, #22269, #12324, #20817, #12843, #22525, #8792, #2387, #14817, #2901, #24750, #16782, #12587, #24484, #4866, #12723, #6834, #6564, #20293, #6692, #20565, #2654, #10868, #22790, #694, #18342, #16396, #20692, #8658, #18868, #24366, #14686, #4753, #18722, #2774, #6442, #14427, #814, #16254, #14937, #13365, #3041, #20960, #5376, #24879, #1340, #21337, #23049, #7465, #11011, #13114, #5136, #3420, #7345, #9049, #16914, #15074, #1194, #22912, #11396, #6958, #18991, #19370, #4997, #9313, #1464, #9436, #17417, #17298, #25380, #12977, #21203, #1075, #13501, #15456, #17031, #23425, #24998, #7086, #21085, #9175 ),
 .UNSPECIFIED., .F., .F. ) 
 B_SPLINE_CURVE_WITH_KNOTS ( ( 3, 2, 2, 2, 2, 2, 2, 2, 2, 2, 2, 2, 2, 2, 2, 2, 2, 2, 2, 2, 2, 2, 2, 2, 2, 2, 2, 2, 2, 2, 2, 2, 2, 2, 2, 2, 2, 2, 2, 2, 2, 2, 2, 2, 2, 2, 2, 2, 2, 2, 2, 2, 2, 2, 2, 2, 2, 2, 2, 2, 3 ),
 ( 0.000000000000000000, 0.01666666666666666644, 0.03333333333333333287, 0.05000000000000000278, 0.06666666666666666574, 0.08333333333333332871, 0.1000000000000000056, 0.1166666666666666685, 0.1333333333333333315, 0.1499999999999999944, 0.1666666666666666574, 0.1833333333333333204, 0.2000000000000000111, 0.2166666666666666741, 0.2333333333333333370, 0.2500000000000000000, 0.2666666666666666630, 0.2833333333333333259, 0.2999999999999999889, 0.3166666666666666519, 0.3333333333333333148, 0.3499999999999999778, 0.3666666666666666408, 0.3833333333333333592, 0.4000000000000000222, 0.4166666666666666852, 0.4333333333333333481, 0.4500000000000000111, 0.4666666666666666741, 0.4833333333333333370, 0.5000000000000000000, 0.5166666666666667185, 0.5333333333333333259, 0.5500000000000000444, 0.5666666666666666519, 0.5833333333333333703, 0.5999999999999999778, 0.6166666666666666963, 0.6333333333333333037, 0.6500000000000000222, 0.6666666666666666297, 0.6833333333333333481, 0.6999999999999999556, 0.7166666666666666741, 0.7333333333333332815, 0.7500000000000000000, 0.7666666666666667185, 0.7833333333333333259, 0.8000000000000000444, 0.8166666666666666519, 0.8333333333333333703, 0.8499999999999999778, 0.8666666666666666963, 0.8833333333333333037, 0.9000000000000000222, 0.9166666666666666297, 0.9333333333333333481, 0.9499999999999999556, 0.9666666666666666741, 0.9833333333333332815, 1.000000000000000000 ),
 .UNSPECIFIED. ) 
 CURVE ( )  GEOMETRIC_REPRESENTATION_ITEM ( )  RATIONAL_B_SPLINE_CURVE ( ( 1.000000000000000000, 0.8660254037844387076, 1.000000000000000000, 0.8660254037844387076, 1.000000000000000000, 0.8660254037844387076, 1.000000000000000000, 0.8660254037844387076, 1.000000000000000000, 0.8660254037844387076, 1.000000000000000000, 0.8660254037844387076, 1.000000000000000000, 0.8660254037844387076, 1.000000000000000000, 0.8660254037844387076, 1.000000000000000000, 0.8660254037844387076, 1.000000000000000000, 0.8660254037844387076, 1.000000000000000000, 0.8660254037844387076, 1.000000000000000000, 0.8660254037844387076, 1.000000000000000000, 0.8660254037844387076, 1.000000000000000000, 0.8660254037844387076, 1.000000000000000000, 0.8660254037844387076, 1.000000000000000000, 0.8660254037844387076, 1.000000000000000000, 0.8660254037844387076, 1.000000000000000000, 0.8660254037844387076, 1.000000000000000000, 0.8660254037844387076, 1.000000000000000000, 0.8660254037844387076, 1.000000000000000000, 0.8660254037844387076, 1.000000000000000000, 0.8660254037844387076, 1.000000000000000000, 0.8660254037844387076, 1.000000000000000000, 0.8660254037844387076, 1.000000000000000000, 0.8660254037844387076, 1.000000000000000000, 0.8660254037844387076, 1.000000000000000000, 0.8660254037844387076, 1.000000000000000000, 0.8660254037844387076, 1.000000000000000000, 0.8660254037844387076, 1.000000000000000000, 0.8660254037844387076, 1.000000000000000000, 0.8660254037844387076, 1.000000000000000000, 0.8660254037844387076, 1.000000000000000000, 0.8660254037844387076, 1.000000000000000000, 0.8660254037844387076, 1.000000000000000000, 0.8660254037844387076, 1.000000000000000000, 0.8660254037844387076, 1.000000000000000000, 0.8660254037844387076, 1.000000000000000000, 0.8660254037844387076, 1.000000000000000000, 0.8660254037844387076, 1.000000000000000000, 0.8660254037844387076, 1.000000000000000000, 0.8660254037844387076, 1.000000000000000000, 0.8660254037844387076, 1.000000000000000000, 0.8660254037844387076, 1.000000000000000000, 0.8660254037844387076, 1.000000000000000000, 0.8660254037844387076, 1.000000000000000000, 0.8660254037844387076, 1.000000000000000000, 0.8660254037844387076, 1.000000000000000000, 0.8660254037844387076, 1.000000000000000000, 0.8660254037844387076, 1.000000000000000000, 0.8660254037844387076, 1.000000000000000000, 0.8660254037844387076, 1.000000000000000000, 0.8660254037844387076, 1.000000000000000000, 0.8660254037844387076, 1.000000000000000000, 0.8660254037844387076, 1.000000000000000000, 0.8660254037844387076, 1.000000000000000000, 0.8660254037844387076, 1.000000000000000000, 0.8660254037844387076, 1.000000000000000000, 0.8660254037844387076, 1.000000000000000000, 0.8660254037844387076, 1.000000000000000000, 0.8660254037844387076, 1.000000000000000000 ) ) 
 REPRESENTATION_ITEM ( '' )  );
#25076=EDGE_LOOP ( 'NONE', ( #12036, #12329, #24887, #18289 ) ) ;
#25088=CARTESIAN_POINT ( 'NONE',  ( -3.756430356249996105, -6.831223922626973533, 0.3281249993854827851 ) ) ;
#25090=VECTOR ( 'NONE', #686, 1000.000000000000000 ) ;
#25091=CARTESIAN_POINT ( 'NONE',  ( 2.672651547586948120E-15, -13.33755215474602984, 4.190624999385483385 ) ) ;
#25097=CYLINDRICAL_SURFACE ( 'NONE', #7970, 4.000000000000000000 ) ;
#25122=CARTESIAN_POINT ( 'NONE',  ( -3.756430356249997882, -11.16877607737301226, 4.565624999385485161 ) ) ;
#25123=CARTESIAN_POINT ( 'NONE',  ( 2.000000000000003997, -5.535898384862238508, 2.268749998770969167 ) ) ;
#25131=CARTESIAN_POINT ( 'NONE',  ( 3.752267015613588906E-15, -4.381197846482986158, 0.1124999999999989342 ) ) ;
#25209=CARTESIAN_POINT ( 'NONE',  ( 2.620986760973688460E-15, -13.61880215351699874, 3.037499999999998757 ) ) ;
#25223=CARTESIAN_POINT ( 'NONE',  ( 3.756430356250002323, -11.16877607737301403, 1.903124999385483740 ) ) ;
#25225=CARTESIAN_POINT ( 'NONE',  ( -3.756430356249995661, -6.831223922626973533, 3.590624999385483740 ) ) ;
#25229=( BOUNDED_CURVE ( )  B_SPLINE_CURVE ( 2, ( #13313, #5597, #25340, #9122, #21541, #25088, #11475, #1670, #17489, #19065, #21045, #7418, #9643, #15400, #23376, #9508, #5461, #1283, #3623, #1148, #19567, #11085, #17626, #11593, #21286, #7550, #17114, #13576, #15021, #23000, #15542, #3367, #17254, #5086, #19447, #15162, #7304, #23132, #13455, #19328, #3505, #5213, #13190, #21160, #11206, #19186, #9267, #25223, #23246, #5329, #11345, #1420, #2191, #6100, #7805, #15668, #7936, #103, #8198, #18153, #15923, #13691, #8076, #25849, #20087, #11976, #4275, #14217, #18016, #5712, #23635, #12113, #21806, #6224, #1808, #11860, #3889, #10152, #14083, #15783, #21667, #3752, #23896, #20216, #5979, #9775, #19708, #4134, #11730, #16055, #227, #16173, #24138, #24019, #22190, #17751, #12247, #2315, #19949, #25724, #23755, #10270, #22048, #25600, #5844, #7683, #13961, #2055, #13828, #1929, #19828, #9892, #17878, #21930, #4010, #10019, #24661, #12641, #350, #6608, #12374 ),
 .UNSPECIFIED., .F., .T. ) 
 B_SPLINE_CURVE_WITH_KNOTS ( ( 3, 2, 2, 2, 2, 2, 2, 2, 2, 2, 2, 2, 2, 2, 2, 2, 2, 2, 2, 2, 2, 2, 2, 2, 2, 2, 2, 2, 2, 2, 2, 2, 2, 2, 2, 2, 2, 2, 2, 2, 2, 2, 2, 2, 2, 2, 2, 2, 2, 2, 2, 2, 2, 2, 2, 2, 2, 2, 2, 2, 3 ),
 ( 0.000000000000000000, 0.01666666666666666644, 0.03333333333333333287, 0.05000000000000000278, 0.06666666666666666574, 0.08333333333333332871, 0.1000000000000000056, 0.1166666666666666685, 0.1333333333333333315, 0.1499999999999999944, 0.1666666666666666574, 0.1833333333333333204, 0.2000000000000000111, 0.2166666666666666741, 0.2333333333333333370, 0.2500000000000000000, 0.2666666666666666630, 0.2833333333333333259, 0.2999999999999999889, 0.3166666666666666519, 0.3333333333333333148, 0.3499999999999999778, 0.3666666666666666408, 0.3833333333333333592, 0.4000000000000000222, 0.4166666666666666852, 0.4333333333333333481, 0.4500000000000000111, 0.4666666666666666741, 0.4833333333333333370, 0.5000000000000000000, 0.5166666666666667185, 0.5333333333333333259, 0.5500000000000000444, 0.5666666666666666519, 0.5833333333333333703, 0.5999999999999999778, 0.6166666666666666963, 0.6333333333333333037, 0.6500000000000000222, 0.6666666666666666297, 0.6833333333333333481, 0.6999999999999999556, 0.7166666666666666741, 0.7333333333333332815, 0.7500000000000000000, 0.7666666666666667185, 0.7833333333333333259, 0.8000000000000000444, 0.8166666666666666519, 0.8333333333333333703, 0.8499999999999999778, 0.8666666666666666963, 0.8833333333333333037, 0.9000000000000000222, 0.9166666666666666297, 0.9333333333333333481, 0.9499999999999999556, 0.9666666666666666741, 0.9833333333333332815, 1.000000000000000000 ),
 .UNSPECIFIED. ) 
 CURVE ( )  GEOMETRIC_REPRESENTATION_ITEM ( )  RATIONAL_B_SPLINE_CURVE ( ( 1.000000000000000000, 0.8660254037844387076, 1.000000000000000000, 0.8660254037844387076, 1.000000000000000000, 0.8660254037844387076, 1.000000000000000000, 0.8660254037844387076, 1.000000000000000000, 0.8660254037844387076, 1.000000000000000000, 0.8660254037844387076, 1.000000000000000000, 0.8660254037844387076, 1.000000000000000000, 0.8660254037844387076, 1.000000000000000000, 0.8660254037844387076, 1.000000000000000000, 0.8660254037844387076, 1.000000000000000000, 0.8660254037844387076, 1.000000000000000000, 0.8660254037844387076, 1.000000000000000000, 0.8660254037844387076, 1.000000000000000000, 0.8660254037844387076, 1.000000000000000000, 0.8660254037844387076, 1.000000000000000000, 0.8660254037844387076, 1.000000000000000000, 0.8660254037844387076, 1.000000000000000000, 0.8660254037844387076, 1.000000000000000000, 0.8660254037844387076, 1.000000000000000000, 0.8660254037844387076, 1.000000000000000000, 0.8660254037844387076, 1.000000000000000000, 0.8660254037844387076, 1.000000000000000000, 0.8660254037844387076, 1.000000000000000000, 0.8660254037844387076, 1.000000000000000000, 0.8660254037844387076, 1.000000000000000000, 0.8660254037844387076, 1.000000000000000000, 0.8660254037844387076, 1.000000000000000000, 0.8660254037844387076, 1.000000000000000000, 0.8660254037844387076, 1.000000000000000000, 0.8660254037844387076, 1.000000000000000000, 0.8660254037844387076, 1.000000000000000000, 0.8660254037844387076, 1.000000000000000000, 0.8660254037844387076, 1.000000000000000000, 0.8660254037844387076, 1.000000000000000000, 0.8660254037844387076, 1.000000000000000000, 0.8660254037844387076, 1.000000000000000000, 0.8660254037844387076, 1.000000000000000000, 0.8660254037844387076, 1.000000000000000000, 0.8660254037844387076, 1.000000000000000000, 0.8660254037844387076, 1.000000000000000000, 0.8660254037844387076, 1.000000000000000000, 0.8660254037844387076, 1.000000000000000000, 0.8660254037844387076, 1.000000000000000000, 0.8660254037844387076, 1.000000000000000000, 0.8660254037844387076, 1.000000000000000000, 0.8660254037844387076, 1.000000000000000000, 0.8660254037844387076, 1.000000000000000000, 0.8660254037844387076, 1.000000000000000000, 0.8660254037844387076, 1.000000000000000000, 0.8660254037844387076, 1.000000000000000000, 0.8660254037844387076, 1.000000000000000000, 0.8660254037844387076, 1.000000000000000000, 0.8660254037844387076, 1.000000000000000000, 0.8660254037844387076, 1.000000000000000000, 0.8660254037844387076, 1.000000000000000000, 0.8660254037844387076, 1.000000000000000000, 0.8660254037844387076, 1.000000000000000000, 0.8660254037844387076, 1.000000000000000000, 0.8660254037844387076, 1.000000000000000000, 0.8660254037844387076, 1.000000000000000000 ) ) 
 REPRESENTATION_ITEM ( '' )  );
#25233=CARTESIAN_POINT ( 'NONE',  ( -3.999999999999996447, -8.999999999999992895, 0.6187499987709670357 ) ) ;
#25253=CARTESIAN_POINT ( 'NONE',  ( -1.878215178124998497, -12.25316411605951927, 0.4406249993854846614 ) ) ;
#25254=CARTESIAN_POINT ( 'NONE',  ( 3.752267015613588906E-15, -4.381197846482986158, 1.856249998770964860 ) ) ;
#25259=CARTESIAN_POINT ( 'NONE',  ( 1.878215178125004048, -5.746835883940462963, 4.265624999385483562 ) ) ;
#25273=CARTESIAN_POINT ( 'NONE',  ( 4.000000000000003553, -8.999999999999992895, 18.00000000000000000 ) ) ;
#25278=( BOUNDED_CURVE ( )  B_SPLINE_CURVE ( 2, ( #25780, #4334, #2118, #12310, #8388, #16380, #11797 ),
 .UNSPECIFIED., .F., .F. ) 
 B_SPLINE_CURVE_WITH_KNOTS ( ( 3, 2, 2, 3 ),
 ( 0.4999999999999997780, 0.5166666666666664964, 0.5333333333333329929, 0.5499999999999997113 ),
 .UNSPECIFIED. ) 
 CURVE ( )  GEOMETRIC_REPRESENTATION_ITEM ( )  RATIONAL_B_SPLINE_CURVE ( ( 1.000000000000001776, 0.8660254037844369313, 1.000000000000000000, 0.8660254037844387076, 1.000000000000000000, 0.8660254037844413721, 0.9999999999999973355 ) ) 
 REPRESENTATION_ITEM ( '' )  );
#25303=EDGE_LOOP ( 'NONE', ( #4036, #21274, #11197, #8134 ) ) ;
#25324=CARTESIAN_POINT ( 'NONE',  ( -3.999999999999996447, -8.999999999999992895, 3.318749998770968102 ) ) ;
#25340=CARTESIAN_POINT ( 'NONE',  ( 1.878215178125004048, -5.746835883940462963, 0.2156249993854816860 ) ) ;
#25341=CARTESIAN_POINT ( 'NONE',  ( 3.756430356250004099, -6.831223922626973533, 4.340624999385483740 ) ) ;
#25369=CARTESIAN_POINT ( 'NONE',  ( -1.878215178124998497, -12.25316411605951927, 1.790624999385481697 ) ) ;
#25370=CARTESIAN_POINT ( 'NONE',  ( 2.000000000000003997, -5.535898384862238508, 2.718749998770968013 ) ) ;
#25373=CARTESIAN_POINT ( 'NONE',  ( 2.000000000000000888, -12.46410161513774817, 3.918749998770967746 ) ) ;
#25375=CARTESIAN_POINT ( 'NONE',  ( 4.000000000000001776, -11.30940107675849760, 2.662499999999997424 ) ) ;
#25380=CARTESIAN_POINT ( 'NONE',  ( 3.756430356250003211, -6.831223922626973533, 4.340624999385483740 ) ) ;
#25383=CARTESIAN_POINT ( 'NONE',  ( 4.000000000000003553, -8.999999999999992895, 3.093749998770968457 ) ) ;
#25417=ORIENTED_EDGE ( 'NONE', *, *, #2225, .F. ) ;
#25443=CARTESIAN_POINT ( 'NONE',  ( 2.000000000000000888, -12.46410161513774817, 3.018749998770966503 ) ) ;
#25467=CARTESIAN_POINT ( 'NONE',  ( 1.878215178125000939, -12.25316411605952283, 3.778124999385484628 ) ) ;
#25503=CARTESIAN_POINT ( 'NONE',  ( 1.878215178125004048, -5.746835883940462963, 2.465624999385483740 ) ) ;
#25504=CARTESIAN_POINT ( 'NONE',  ( 2.000000000000000888, -12.46410161513774817, 0.7687499987709678351 ) ) ;
#25511=CARTESIAN_POINT ( 'NONE',  ( 2.620986760973688460E-15, -13.61880215351699874, 2.137499999999999734 ) ) ;
#25548=CARTESIAN_POINT ( 'NONE',  ( 4.000000000000003553, -8.999999999999992895, 3.993749998770966592 ) ) ;
#25549=AXIS2_PLACEMENT_3D ( 'NONE', #1747, #21995, #11922 ) ;
#25600=CARTESIAN_POINT ( 'NONE',  ( -3.756430356249997438, -11.16877607737301048, 4.003124999385478056 ) ) ;
#25608=DIRECTION ( 'NONE',  ( -0.000000000000000000, -0.000000000000000000, -1.000000000000000000 ) ) ;
#25610=DIRECTION ( 'NONE',  ( -1.000000000000000000, 0.000000000000000000, 0.000000000000000000 ) ) ;
#25632=ORIENTED_EDGE ( 'NONE', *, *, #7937, .F. ) ;
#25637=CARTESIAN_POINT ( 'NONE',  ( 2.672651547586948120E-15, -13.33755215474602984, 2.728124999385481253 ) ) ;
#25638=CARTESIAN_POINT ( 'NONE',  ( 3.752267015613588906E-15, -4.381197846482986158, 1.406249998770964904 ) ) ;
#25643=CARTESIAN_POINT ( 'NONE',  ( 4.000000000000001776, -11.30940107675849760, 1.312499999999998224 ) ) ;
#25657=ORIENTED_EDGE ( 'NONE', *, *, #15600, .F. ) ;
#25662=ORIENTED_EDGE ( 'NONE', *, *, #20514, .T. ) ;
#25669=CARTESIAN_POINT ( 'NONE',  ( -3.756430356249995661, -6.831223922626973533, 1.340624999385481075 ) ) ;
#25675=CARTESIAN_POINT ( 'NONE',  ( 2.620986760973688460E-15, -13.61880215351699874, 3.487499999999998934 ) ) ;
#25724=CARTESIAN_POINT ( 'NONE',  ( 3.735045420075836212E-15, -4.662447845253954171, 3.853124999385482585 ) ) ;
#25729=DIRECTION ( 'NONE',  ( -1.000000000000000000, 0.000000000000000000, 0.000000000000000000 ) ) ;
#25740=ORIENTED_EDGE ( 'NONE', *, *, #15408, .F. ) ;
#25755=CARTESIAN_POINT ( 'NONE',  ( -3.756430356249996994, -8.999999999999992895, 2.615624999385480987 ) ) ;
#25756=CARTESIAN_POINT ( 'NONE',  ( -1.999999999999995781, -5.535898384862237620, 3.243749998770965703 ) ) ;
#25762=CARTESIAN_POINT ( 'NONE',  ( 2.000000000000003997, -5.535898384862238508, 2.774999999999999467 ) ) ;
#25772=VERTEX_POINT ( 'NONE', #24988 ) ;
#25780=CARTESIAN_POINT ( 'NONE',  ( 4.000000000000003553, -8.999999999999992895, 2.643749998770966059 ) ) ;
#25784=CARTESIAN_POINT ( 'NONE',  ( 2.672651547586948120E-15, -13.33755215474602984, 0.5906249993854855163 ) ) ;
#25831=VECTOR ( 'NONE', #5262, 1000.000000000000000 ) ;
#25840=ORIENTED_EDGE ( 'NONE', *, *, #12249, .T. ) ;
#25849=CARTESIAN_POINT ( 'NONE',  ( 3.735045420075836212E-15, -4.662447845253954171, 2.503124999385483385 ) ) ;
#25858=CARTESIAN_POINT ( 'NONE',  ( 3.469446951953614189E-15, -8.999999999999992895, 18.00000000000000000 ) ) ;
#25901=COLOUR_RGB('Sky Blue',0.24,0.69,0.87);
#25902=FILL_AREA_STYLE_COLOUR('',#25901);
#25903=FILL_AREA_STYLE('',(#25902));
#25904=SURFACE_STYLE_FILL_AREA(#25903);
#25905=SURFACE_SIDE_STYLE('',(#25904));
#25906=SURFACE_STYLE_USAGE(.BOTH.,#25905);
#25907=PRESENTATION_STYLE_ASSIGNMENT((#25906));
ENDSEC;
END-ISO-10303-21;
